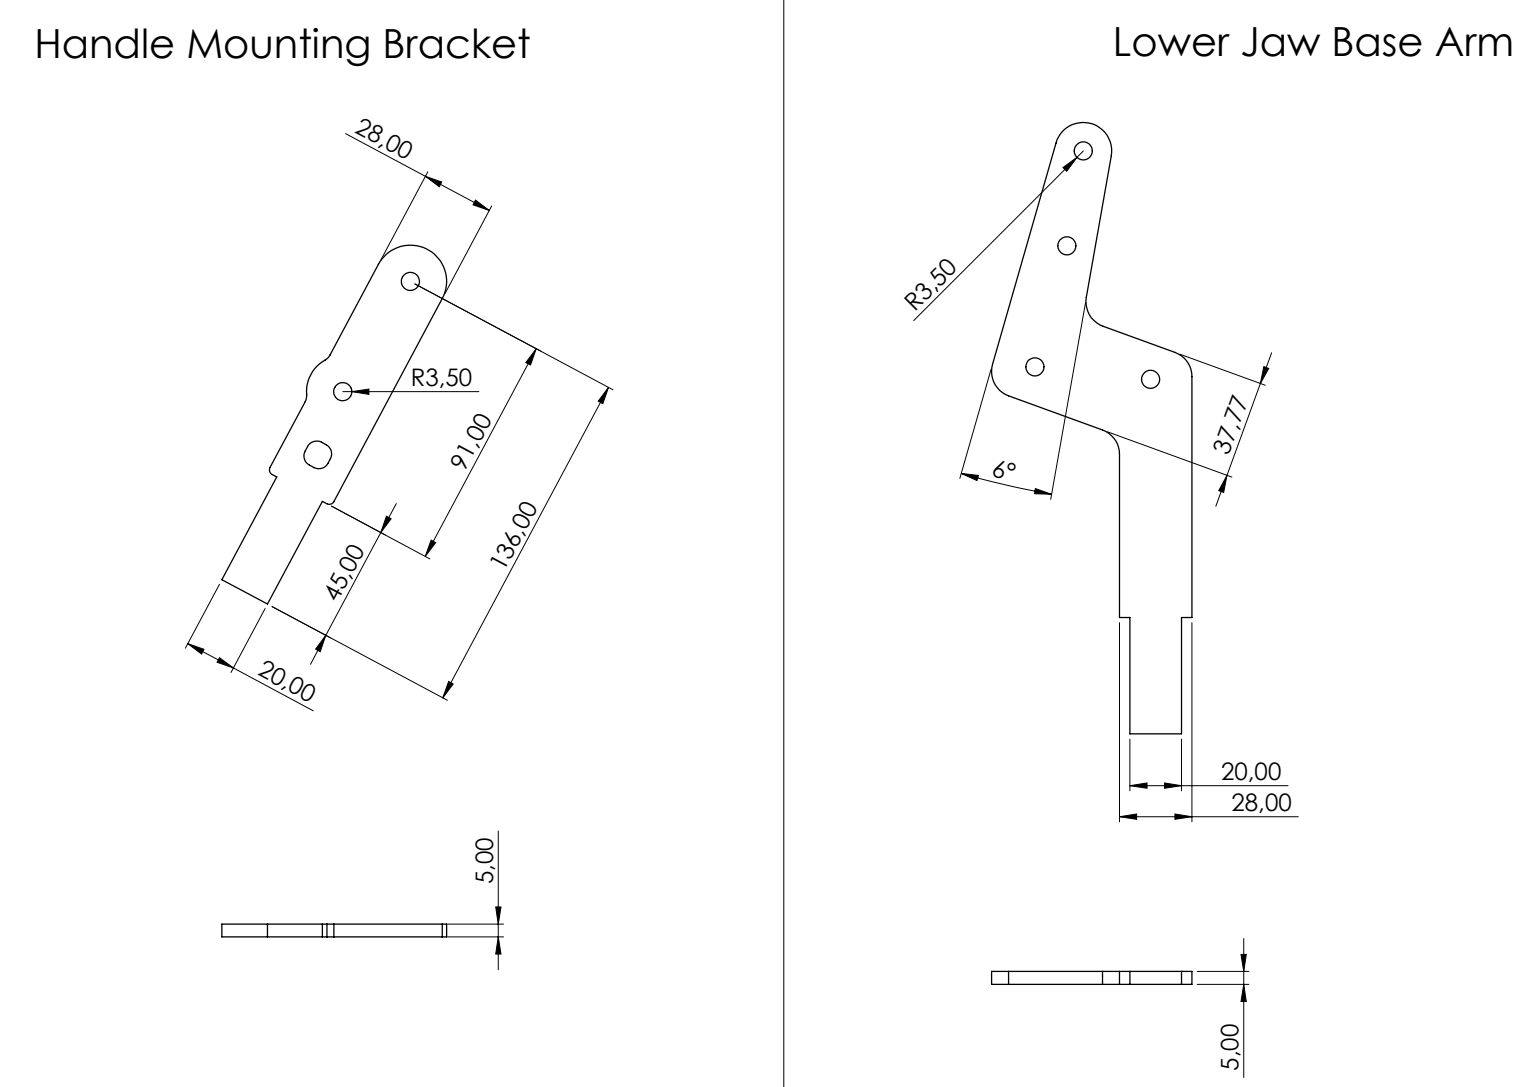
ISO-10303-21;
HEADER;
FILE_DESCRIPTION (('STEP AP214'),
    '1' );
FILE_NAME ('Handle Mounting Bracket.step',
    '2026-10-06T08:24:18',
    ( '' ),
    ( '' ),
    'SwSTEP 2.0',
    'SolidWorks 2020',
    '' );
FILE_SCHEMA (( 'AUTOMOTIVE_DESIGN' ));
ENDSEC;

DATA;
#12=AXIS2_PLACEMENT_3D ( 'NONE', #3802, #4074, #7998 ) ;
#21=PLANE ( 'NONE',  #9517 ) ;
#25=AXIS2_PLACEMENT_3D ( 'NONE', #9737, #2431, #8928 ) ;
#36=EDGE_CURVE ( 'NONE', #6471, #8445, #5902, .T. ) ;
#38=ORIENTED_EDGE ( 'NONE', *, *, #7830, .T. ) ;
#56=VERTEX_POINT ( 'NONE', #5109 ) ;
#58=CARTESIAN_POINT ( 'NONE',  ( -101.0297452788102817, -7.500000000000000000, -342.4231267849074811 ) ) ;
#62=ORIENTED_EDGE ( 'NONE', *, *, #1562, .F. ) ;
#65=DIRECTION ( 'NONE',  ( -0.8820010751365716661, 0.000000000000000000, -0.4712473909295749053 ) ) ;
#66=CARTESIAN_POINT ( 'NONE',  ( -87.43749534091338660, -7.500000000000000000, -367.8627987905216514 ) ) ;
#77=VECTOR ( 'NONE', #6835, 1000.000000000000000 ) ;
#85=DIRECTION ( 'NONE',  ( 0.000000000000000000, -1.000000000000000000, 0.000000000000000000 ) ) ;
#86=VECTOR ( 'NONE', #9017, 1000.000000000000000 ) ;
#96=CARTESIAN_POINT ( 'NONE',  ( -102.0103468492230547, -7.500000000000000000, -289.6591388711787545 ) ) ;
#120=CARTESIAN_POINT ( 'NONE',  ( -77.67426137820133647, -2.500000000000000000, -345.8174414091573681 ) ) ;
#132=DIRECTION ( 'NONE',  ( -0.4712473909295827323, 0.000000000000000000, 0.8820010751365675583 ) ) ;
#186=EDGE_LOOP ( 'NONE', ( #828, #1603, #62, #6851 ) ) ;
#211=VECTOR ( 'NONE', #3924, 1000.000000000000000 ) ;
#216=DIRECTION ( 'NONE',  ( 0.4712473909295827323, 0.000000000000000000, -0.8820010751365675583 ) ) ;
#230=LINE ( 'NONE', #8685, #4617 ) ;
#241=DIRECTION ( 'NONE',  ( 0.8820010751365678914, 0.000000000000000000, 0.4712473909295818442 ) ) ;
#251=CIRCLE ( 'NONE', #9352, 3.500000000000003997 ) ;
#257=ORIENTED_EDGE ( 'NONE', *, *, #493, .F. ) ;
#269=VERTEX_POINT ( 'NONE', #6973 ) ;
#290=CARTESIAN_POINT ( 'NONE',  ( -59.08872748607741698, -7.500000000000000000, -420.9212224720619702 ) ) ;
#304=ORIENTED_EDGE ( 'NONE', *, *, #2921, .F. ) ;
#306=VERTEX_POINT ( 'NONE', #406 ) ;
#316=AXIS2_PLACEMENT_3D ( 'NONE', #10425, #6337, #7104 ) ;
#320=VERTEX_POINT ( 'NONE', #10191 ) ;
#324=CARTESIAN_POINT ( 'NONE',  ( -99.26574312853713877, -7.500000000000000000, -341.4806320030483562 ) ) ;
#354=ORIENTED_EDGE ( 'NONE', *, *, #10397, .T. ) ;
#363=EDGE_CURVE ( 'NONE', #1218, #8202, #3035, .T. ) ;
#389=AXIS2_PLACEMENT_3D ( 'NONE', #10091, #3429, #953 ) ;
#390=ORIENTED_EDGE ( 'NONE', *, *, #6600, .F. ) ;
#392=CARTESIAN_POINT ( 'NONE',  ( -79.04021210711869116, -7.500000000000000000, -328.4066924704651456 ) ) ;
#393=CARTESIAN_POINT ( 'NONE',  ( -77.77979771402830522, -2.500000000000000000, -385.9384419754180158 ) ) ;
#394=ORIENTED_EDGE ( 'NONE', *, *, #6640, .T. ) ;
#404=DIRECTION ( 'NONE',  ( 0.000000000000000000, -1.000000000000000000, 0.000000000000000000 ) ) ;
#406=CARTESIAN_POINT ( 'NONE',  ( -79.74686404004059170, -2.500000000000000000, -383.9321052860355508 ) ) ;
#416=ORIENTED_EDGE ( 'NONE', *, *, #9414, .F. ) ;
#422=EDGE_CURVE ( 'NONE', #306, #9067, #9592, .T. ) ;
#425=CARTESIAN_POINT ( 'NONE',  ( -84.02975002432511076, -2.500000000000000000, -342.4104245220563030 ) ) ;
#426=AXIS2_PLACEMENT_3D ( 'NONE', #4824, #7296, #1375 ) ;
#432=EDGE_CURVE ( 'NONE', #700, #6716, #7233, .T. ) ;
#437=EDGE_CURVE ( 'NONE', #3828, #7650, #10190, .T. ) ;
#465=( LENGTH_UNIT ( ) NAMED_UNIT ( * ) SI_UNIT ( .MILLI., .METRE. ) );
#473=ORIENTED_EDGE ( 'NONE', *, *, #1711, .T. ) ;
#474=CIRCLE ( 'NONE', #7341, 4.000000000000008882 ) ;
#476=CARTESIAN_POINT ( 'NONE',  ( -78.61675616006050404, -7.500000000000000000, -344.0534392588842252 ) ) ;
#486=CARTESIAN_POINT ( 'NONE',  ( -79.74686404004059170, -7.500000000000000000, -383.9321052860355508 ) ) ;
#493=EDGE_CURVE ( 'NONE', #7563, #4961, #4707, .T. ) ;
#509=EDGE_LOOP ( 'NONE', ( #4732, #10118, #10336, #1157 ) ) ;
#512=AXIS2_PLACEMENT_3D ( 'NONE', #1643, #10610, #2448 ) ;
#520=AXIS2_PLACEMENT_3D ( 'NONE', #3309, #8355, #7553 ) ;
#529=CIRCLE ( 'NONE', #6531, 14.00000000000000888 ) ;
#531=STYLED_ITEM ( 'NONE', ( #3235 ), #1856 ) ;
#532=LINE ( 'NONE', #2793, #8706 ) ;
#536=CARTESIAN_POINT ( 'NONE',  ( -86.49427212956700828, -7.500000000000000000, -350.5299153184531633 ) ) ;
#568=EDGE_CURVE ( 'NONE', #9067, #6664, #8056, .T. ) ;
#581=VECTOR ( 'NONE', #10244, 1000.000000000000000 ) ;
#592=CIRCLE ( 'NONE', #7969, 4.000000000000009770 ) ;
#594=DIRECTION ( 'NONE',  ( 0.000000000000000000, 1.000000000000000000, -0.000000000000000000 ) ) ;
#636=CARTESIAN_POINT ( 'NONE',  ( -72.90663470096859555, -2.500000000000000000, -371.7168990827444190 ) ) ;
#640=FACE_BOUND ( 'NONE', #5175, .T. ) ;
#665=CARTESIAN_POINT ( 'NONE',  ( -79.31727611502927289, -2.500000000000000000, -351.2304352734219606 ) ) ;
#667=PRODUCT_DEFINITION_CONTEXT ( 'detailed design', #7443, 'design' ) ;
#670=EDGE_CURVE ( 'NONE', #1738, #2124, #8074, .T. ) ;
#681=CIRCLE ( 'NONE', #10112, 3.499999999999997335 ) ;
#696=CYLINDRICAL_SURFACE ( 'NONE', #389, 1.999999999999980238 ) ;
#700=VERTEX_POINT ( 'NONE', #818 ) ;
#703=DIRECTION ( 'NONE',  ( -0.4712473909295803454, 0.000000000000000000, 0.8820010751365688906 ) ) ;
#709=CARTESIAN_POINT ( 'NONE',  ( -119.6503683519543983, -2.500000000000000000, -299.0840866897705155 ) ) ;
#713=( LENGTH_UNIT ( ) NAMED_UNIT ( * ) SI_UNIT ( .MILLI., .METRE. ) );
#730=DIRECTION ( 'NONE',  ( 0.4712473909295803454, 0.000000000000000000, -0.8820010751365688906 ) ) ;
#750=ORIENTED_EDGE ( 'NONE', *, *, #4566, .F. ) ;
#751=ORIENTED_EDGE ( 'NONE', *, *, #437, .F. ) ;
#773=DIRECTION ( 'NONE',  ( 0.000000000000000000, 1.000000000000000000, -0.000000000000000000 ) ) ;
#778=ORIENTED_EDGE ( 'NONE', *, *, #2712, .F. ) ;
#789=FACE_OUTER_BOUND ( 'NONE', #10203, .T. ) ;
#795=CARTESIAN_POINT ( 'NONE',  ( -72.90663470096859555, -2.500000000000000000, -371.7168990827444190 ) ) ;
#803=ORIENTED_EDGE ( 'NONE', *, *, #2276, .T. ) ;
#807=CARTESIAN_POINT ( 'NONE',  ( -98.44423576012317767, -2.500000000000000000, -338.7741350709160315 ) ) ;
#812=CARTESIAN_POINT ( 'NONE',  ( -76.33371517498638070, -2.500000000000000000, -329.2281998388791635 ) ) ;
#818=CARTESIAN_POINT ( 'NONE',  ( -87.43749534091338660, -2.500000000000000000, -367.8627987905216514 ) ) ;
#826=EDGE_LOOP ( 'NONE', ( #4070, #3945, #7397, #4001, #5011, #9817, #8400, #8877 ) ) ;
#828=ORIENTED_EDGE ( 'NONE', *, *, #8175, .T. ) ;
#862=DIRECTION ( 'NONE',  ( 0.8820010751365675583, 0.000000000000000000, 0.4712473909295827323 ) ) ;
#875=ORIENTED_EDGE ( 'NONE', *, *, #1881, .F. ) ;
#889=DIRECTION ( 'NONE',  ( 0.000000000000000000, -1.000000000000000000, 0.000000000000000000 ) ) ;
#895=CYLINDRICAL_SURFACE ( 'NONE', #7546, 13.99999999999999645 ) ;
#902=DIRECTION ( 'NONE',  ( -0.4712473909295827323, 0.000000000000000000, 0.8820010751365675583 ) ) ;
#912=LINE ( 'NONE', #4202, #6782 ) ;
#916=DIRECTION ( 'NONE',  ( 0.000000000000000000, 1.000000000000000000, -0.000000000000000000 ) ) ;
#932=VERTEX_POINT ( 'NONE', #9124 ) ;
#946=ORIENTED_EDGE ( 'NONE', *, *, #9826, .T. ) ;
#948=DIRECTION ( 'NONE',  ( 0.000000000000000000, -1.000000000000000000, 0.000000000000000000 ) ) ;
#953=DIRECTION ( 'NONE',  ( -0.4712473909295860630, 0.000000000000000000, 0.8820010751365656709 ) ) ;
#968=DIRECTION ( 'NONE',  ( 0.000000000000000000, 1.000000000000000000, -0.000000000000000000 ) ) ;
#974=CARTESIAN_POINT ( 'NONE',  ( -46.74071243416547361, -2.500000000000000000, -414.3237589990478114 ) ) ;
#977=EDGE_CURVE ( 'NONE', #5188, #932, #681, .T. ) ;
#1011=DIRECTION ( 'NONE',  ( 0.8820010751365716661, 0.000000000000000000, 0.4712473909295749053 ) ) ;
#1034=CARTESIAN_POINT ( 'NONE',  ( -72.90663470096859555, -7.500000000000000000, -371.7168990827444190 ) ) ;
#1035=AXIS2_PLACEMENT_3D ( 'NONE', #974, #1730, #862 ) ;
#1040=AXIS2_PLACEMENT_3D ( 'NONE', #7215, #5321, #6238 ) ;
#1048=ORIENTED_EDGE ( 'NONE', *, *, #5342, .F. ) ;
#1052=VERTEX_POINT ( 'NONE', #6047 ) ;
#1093=CIRCLE ( 'NONE', #4515, 5.000000000000008882 ) ;
#1106=CARTESIAN_POINT ( 'NONE',  ( -82.18980308971114823, -2.500000000000000000, -388.2946789300659134 ) ) ;
#1119=ORIENTED_EDGE ( 'NONE', *, *, #7066, .F. ) ;
#1126=LINE ( 'NONE', #2795, #10298 ) ;
#1128=CARTESIAN_POINT ( 'NONE',  ( -72.90663470096859555, -7.500000000000000000, -371.7168990827444190 ) ) ;
#1140=ORIENTED_EDGE ( 'NONE', *, *, #4953, .T. ) ;
#1152=ORIENTED_EDGE ( 'NONE', *, *, #4382, .T. ) ;
#1157=ORIENTED_EDGE ( 'NONE', *, *, #2791, .F. ) ;
#1167=CIRCLE ( 'NONE', #7689, 5.000000000000006217 ) ;
#1170=ORIENTED_EDGE ( 'NONE', *, *, #2276, .F. ) ;
#1177=FACE_OUTER_BOUND ( 'NONE', #10616, .T. ) ;
#1190=CARTESIAN_POINT ( 'NONE',  ( -89.32175647514451100, -2.500000000000000000, -345.2379088676337915 ) ) ;
#1197=LINE ( 'NONE', #8604, #4995 ) ;
#1200=CARTESIAN_POINT ( 'NONE',  ( -79.31727611502927289, -7.500000000000000000, -351.2304352734219606 ) ) ;
#1211=LINE ( 'NONE', #10139, #9926 ) ;
#1218=VERTEX_POINT ( 'NONE', #6075 ) ;
#1221=DIRECTION ( 'NONE',  ( 0.000000000000000000, 1.000000000000000000, -0.000000000000000000 ) ) ;
#1257=ORIENTED_EDGE ( 'NONE', *, *, #2987, .F. ) ;
#1266=AXIS2_PLACEMENT_3D ( 'NONE', #9096, #5703, #2433 ) ;
#1276=AXIS2_PLACEMENT_3D ( 'NONE', #6620, #9898, #9257 ) ;
#1286=PLANE ( 'NONE',  #4156 ) ;
#1301=VERTEX_POINT ( 'NONE', #6124 ) ;
#1308=EDGE_LOOP ( 'NONE', ( #7865, #5755, #3971, #875 ) ) ;
#1317=CARTESIAN_POINT ( 'NONE',  ( -34.39269738225353024, -2.500000000000000000, -407.7262955260336525 ) ) ;
#1327=FACE_OUTER_BOUND ( 'NONE', #5253, .T. ) ;
#1341=CARTESIAN_POINT ( 'NONE',  ( -119.6503683519543983, -7.500000000000000000, -299.0840866897705155 ) ) ;
#1344=CARTESIAN_POINT ( 'NONE',  ( -78.52752440735136474, -2.500000000000000000, -384.5389737553005034 ) ) ;
#1351=DIRECTION ( 'NONE',  ( -0.8820010751365675583, 0.000000000000000000, -0.4712473909295827323 ) ) ;
#1361=AXIS2_PLACEMENT_3D ( 'NONE', #9213, #7589, #5809 ) ;
#1363=ORIENTED_EDGE ( 'NONE', *, *, #977, .T. ) ;
#1364=CARTESIAN_POINT ( 'NONE',  ( -79.31727611502927289, -2.500000000000000000, -351.2304352734219606 ) ) ;
#1373=VERTEX_POINT ( 'NONE', #1341 ) ;
#1375=DIRECTION ( 'NONE',  ( -0.8820010751365678914, 0.000000000000000000, -0.4712473909295818442 ) ) ;
#1380=CARTESIAN_POINT ( 'NONE',  ( -86.86306229143158930, -2.500000000000000000, -370.6132103076870976 ) ) ;
#1384=FACE_OUTER_BOUND ( 'NONE', #4703, .T. ) ;
#1418=VERTEX_POINT ( 'NONE', #6174 ) ;
#1424=CARTESIAN_POINT ( 'NONE',  ( -80.80421425739181984, -2.500000000000000000, -329.3491872523243842 ) ) ;
#1429=ORIENTED_EDGE ( 'NONE', *, *, #5752, .F. ) ;
#1432=ORIENTED_EDGE ( 'NONE', *, *, #6163, .F. ) ;
#1457=AXIS2_PLACEMENT_3D ( 'NONE', #5077, #10617, #4173 ) ;
#1460=PRODUCT_CONTEXT ( 'NONE', #2761, 'mechanical' ) ;
#1467=ORIENTED_EDGE ( 'NONE', *, *, #5835, .F. ) ;
#1477=ADVANCED_FACE ( 'NONE', ( #4789 ), #7258, .F. ) ;
#1480=DIRECTION ( 'NONE',  ( -0.8820010751365675583, 0.000000000000000000, -0.4712473909295827323 ) ) ;
#1481=ORIENTED_EDGE ( 'NONE', *, *, #1562, .T. ) ;
#1485=ADVANCED_FACE ( 'NONE', ( #9729 ), #3975, .T. ) ;
#1493=ORIENTED_EDGE ( 'NONE', *, *, #432, .F. ) ;
#1514=CARTESIAN_POINT ( 'NONE',  ( -84.02975002432511076, -2.500000000000000000, -342.4104245220563030 ) ) ;
#1519=VERTEX_POINT ( 'NONE', #9321 ) ;
#1525=EDGE_LOOP ( 'NONE', ( #4822, #7801, #3032, #3409 ) ) ;
#1535=ADVANCED_FACE ( 'NONE', ( #10169 ), #9270, .T. ) ;
#1547=CARTESIAN_POINT ( 'NONE',  ( -80.80421425739181984, -7.500000000000000000, -329.3491872523243842 ) ) ;
#1549=VECTOR ( 'NONE', #3392, 1000.000000000000000 ) ;
#1561=ORIENTED_EDGE ( 'NONE', *, *, #568, .T. ) ;
#1562=EDGE_CURVE ( 'NONE', #320, #8561, #2812, .T. ) ;
#1593=VECTOR ( 'NONE', #8757, 1000.000000000000000 ) ;
#1603=ORIENTED_EDGE ( 'NONE', *, *, #9616, .T. ) ;
#1607=CARTESIAN_POINT ( 'NONE',  ( -83.90876261087991850, -7.500000000000000000, -346.8809236044617137 ) ) ;
#1619=PLANE ( 'NONE',  #3401 ) ;
#1625=( NAMED_UNIT ( * ) PLANE_ANGLE_UNIT ( ) SI_UNIT ( $, .RADIAN. ) );
#1630=VECTOR ( 'NONE', #3515, 1000.000000000000000 ) ;
#1631=CIRCLE ( 'NONE', #1276, 5.000000000000008882 ) ;
#1643=CARTESIAN_POINT ( 'NONE',  ( -82.18980308971114823, -7.500000000000000000, -388.2946789300659134 ) ) ;
#1671=EDGE_CURVE ( 'NONE', #9606, #10567, #2305, .T. ) ;
#1677=ORIENTED_EDGE ( 'NONE', *, *, #10150, .F. ) ;
#1685=CYLINDRICAL_SURFACE ( 'NONE', #3076, 1.999999999999998224 ) ;
#1689=VERTEX_POINT ( 'NONE', #3721 ) ;
#1701=CARTESIAN_POINT ( 'NONE',  ( -82.14476046060677561, -2.500000000000000000, -345.9384288226025888 ) ) ;
#1702=CARTESIAN_POINT ( 'NONE',  ( -69.81963093799060971, -7.500000000000000000, -370.0675332144908793 ) ) ;
#1711=EDGE_CURVE ( 'NONE', #4107, #7563, #6183, .T. ) ;
#1718=CARTESIAN_POINT ( 'NONE',  ( -78.09771732525952359, -7.500000000000000000, -330.1706946207383453 ) ) ;
#1729=SURFACE_SIDE_STYLE ('',( #3344 ) ) ;
#1730=DIRECTION ( 'NONE',  ( 0.000000000000000000, 1.000000000000000000, -0.000000000000000000 ) ) ;
#1738=VERTEX_POINT ( 'NONE', #7855 ) ;
#1749=CARTESIAN_POINT ( 'NONE',  ( -34.39269738225353024, -7.500000000000000000, -407.7262955260336525 ) ) ;
#1751=CYLINDRICAL_SURFACE ( 'NONE', #1457, 3.499999999999997335 ) ;
#1755=CIRCLE ( 'NONE', #3123, 3.500000000000003997 ) ;
#1757=CARTESIAN_POINT ( 'NONE',  ( -34.39269738225353024, -2.500000000000000000, -407.7262955260336525 ) ) ;
#1765=VECTOR ( 'NONE', #5247, 1000.000000000000000 ) ;
#1774=EDGE_CURVE ( 'NONE', #9600, #5739, #2422, .T. ) ;
#1799=CIRCLE ( 'NONE', #4031, 14.00000000000000888 ) ;
#1804=AXIS2_PLACEMENT_3D ( 'NONE', #6758, #9066, #9923 ) ;
#1814=ORIENTED_EDGE ( 'NONE', *, *, #6930, .T. ) ;
#1818=DIRECTION ( 'NONE',  ( -0.8820010751365675583, 0.000000000000000000, -0.4712473909295825103 ) ) ;
#1822=CARTESIAN_POINT ( 'NONE',  ( -119.6503683519543983, -2.500000000000000000, -299.0840866897705155 ) ) ;
#1847=ORIENTED_EDGE ( 'NONE', *, *, #7977, .F. ) ;
#1856=MANIFOLD_SOLID_BREP ( 'Stock-MAS-686-1', #5554 ) ;
#1869=EDGE_CURVE ( 'NONE', #932, #4003, #7480, .T. ) ;
#1874=DIRECTION ( 'NONE',  ( 0.000000000000000000, 1.000000000000000000, -0.000000000000000000 ) ) ;
#1881=EDGE_CURVE ( 'NONE', #1689, #1519, #4653, .T. ) ;
#1897=FACE_OUTER_BOUND ( 'NONE', #2231, .T. ) ;
#1911=LINE ( 'NONE', #5984, #3303 ) ;
#1915=DIRECTION ( 'NONE',  ( 0.000000000000000000, -1.000000000000000000, 0.000000000000000000 ) ) ;
#1919=DIRECTION ( 'NONE',  ( 0.000000000000000000, 1.000000000000000000, -0.000000000000000000 ) ) ;
#1943=ADVANCED_FACE ( 'NONE', ( #2115 ), #6140, .F. ) ;
#1950=UNCERTAINTY_MEASURE_WITH_UNIT (LENGTH_MEASURE( 1.000000000000000082E-05 ), #10396, 'distance_accuracy_value', 'NONE');
#1979=LINE ( 'NONE', #6154, #1765 ) ;
#1995=EDGE_CURVE ( 'NONE', #1689, #8136, #1197, .T. ) ;
#2061=AXIS2_PLACEMENT_3D ( 'NONE', #6419, #7392, #730 ) ;
#2064=CIRCLE ( 'NONE', #1035, 3.499999999999997335 ) ;
#2077=FILL_AREA_STYLE ('',( #4544 ) ) ;
#2082=EDGE_CURVE ( 'NONE', #56, #4107, #2972, .T. ) ;
#2084=ORIENTED_EDGE ( 'NONE', *, *, #8293, .F. ) ;
#2089=DIRECTION ( 'NONE',  ( -0.4712473909295860630, 0.000000000000000000, 0.8820010751365656709 ) ) ;
#2103=CARTESIAN_POINT ( 'NONE',  ( -80.80421425739181984, -2.500000000000000000, -329.3491872523243842 ) ) ;
#2115=FACE_OUTER_BOUND ( 'NONE', #7123, .T. ) ;
#2117=ORIENTED_EDGE ( 'NONE', *, *, #1671, .F. ) ;
#2124=VERTEX_POINT ( 'NONE', #5758 ) ;
#2166=ORIENTED_EDGE ( 'NONE', *, *, #7924, .T. ) ;
#2177=ORIENTED_EDGE ( 'NONE', *, *, #2731, .F. ) ;
#2192=DIRECTION ( 'NONE',  ( 0.4712473909295827323, 0.000000000000000000, -0.8820010751365675583 ) ) ;
#2209=CARTESIAN_POINT ( 'NONE',  ( -102.0103468492230547, -2.500000000000000000, -289.6591388711787545 ) ) ;
#2222=CIRCLE ( 'NONE', #6884, 4.000000000000009770 ) ;
#2231=EDGE_LOOP ( 'NONE', ( #5461, #1677, #4432, #9762 ) ) ;
#2261=DIRECTION ( 'NONE',  ( -0.8820010751365675583, 0.000000000000000000, -0.4712473909295827323 ) ) ;
#2267=CIRCLE ( 'NONE', #8270, 3.499999999999997335 ) ;
#2276=EDGE_CURVE ( 'NONE', #8515, #5739, #3659, .T. ) ;
#2284=CARTESIAN_POINT ( 'NONE',  ( -72.90663470096859555, -2.500000000000000000, -371.7168990827444190 ) ) ;
#2302=CARTESIAN_POINT ( 'NONE',  ( -46.74071243416547361, -7.500000000000000000, -414.3237589990478114 ) ) ;
#2305=CIRCLE ( 'NONE', #1040, 3.500000000000003997 ) ;
#2340=ORIENTED_EDGE ( 'NONE', *, *, #36, .F. ) ;
#2350=LINE ( 'NONE', #8952, #5308 ) ;
#2353=EDGE_CURVE ( 'NONE', #56, #5548, #474, .T. ) ;
#2363=FACE_OUTER_BOUND ( 'NONE', #186, .T. ) ;
#2370=CARTESIAN_POINT ( 'NONE',  ( -34.39269738225353024, -2.500000000000000000, -407.7262955260336525 ) ) ;
#2422=CIRCLE ( 'NONE', #7053, 1.999999999999998224 ) ;
#2431=DIRECTION ( 'NONE',  ( 0.000000000000000000, -1.000000000000000000, 0.000000000000000000 ) ) ;
#2433=DIRECTION ( 'NONE',  ( -0.8820010751365675583, 0.000000000000000000, -0.4712473909295825103 ) ) ;
#2448=DIRECTION ( 'NONE',  ( 0.4885878099338311631, 0.000000000000000000, 0.8725147288063752615 ) ) ;
#2460=LINE ( 'NONE', #96, #9501 ) ;
#2479=LINE ( 'NONE', #807, #4117 ) ;
#2497=ORIENTED_EDGE ( 'NONE', *, *, #7977, .T. ) ;
#2505=DIRECTION ( 'NONE',  ( 0.8820010751365653379, 0.000000000000000000, 0.4712473909295871732 ) ) ;
#2527=ORIENTED_EDGE ( 'NONE', *, *, #6205, .T. ) ;
#2561=ORIENTED_EDGE ( 'NONE', *, *, #1869, .F. ) ;
#2565=DIRECTION ( 'NONE',  ( 0.000000000000000000, -1.000000000000000000, 0.000000000000000000 ) ) ;
#2567=VECTOR ( 'NONE', #5886, 1000.000000000000000 ) ;
#2570=FACE_OUTER_BOUND ( 'NONE', #1525, .T. ) ;
#2573=CARTESIAN_POINT ( 'NONE',  ( -43.65370867118748777, -7.500000000000000000, -412.6743931307942717 ) ) ;
#2575=ADVANCED_FACE ( 'NONE', ( #9730, #3928, #7207, #6557 ), #1619, .F. ) ;
#2588=DIRECTION ( 'NONE',  ( -0.4712473909295827323, 0.000000000000000000, 0.8820010751365675583 ) ) ;
#2599=CARTESIAN_POINT ( 'NONE',  ( -77.67426137820133647, -7.500000000000000000, -345.8174414091573681 ) ) ;
#2607=VERTEX_POINT ( 'NONE', #58 ) ;
#2615=ORIENTED_EDGE ( 'NONE', *, *, #4909, .T. ) ;
#2644=VECTOR ( 'NONE', #4287, 1000.000000000000000 ) ;
#2657=FACE_OUTER_BOUND ( 'NONE', #6360, .T. ) ;
#2669=VECTOR ( 'NONE', #5090, 1000.000000000000000 ) ;
#2671=ORIENTED_EDGE ( 'NONE', *, *, #9703, .T. ) ;
#2686=LINE ( 'NONE', #5037, #10175 ) ;
#2689=ORIENTED_EDGE ( 'NONE', *, *, #2987, .T. ) ;
#2694=LINE ( 'NONE', #6012, #1549 ) ;
#2698=EDGE_CURVE ( 'NONE', #8515, #2607, #8883, .T. ) ;
#2704=CARTESIAN_POINT ( 'NONE',  ( -78.61675616006050404, -2.500000000000000000, -344.0534392588842252 ) ) ;
#2712=EDGE_CURVE ( 'NONE', #9606, #7707, #9555, .T. ) ;
#2731=EDGE_CURVE ( 'NONE', #8080, #700, #1167, .T. ) ;
#2761=APPLICATION_CONTEXT ( 'automotive_design' ) ;
#2791=EDGE_CURVE ( 'NONE', #3089, #6862, #532, .T. ) ;
#2793=CARTESIAN_POINT ( 'NONE',  ( -78.61675616006050404, -2.500000000000000000, -344.0534392588842252 ) ) ;
#2795=CARTESIAN_POINT ( 'NONE',  ( -76.33371517498638070, -7.500000000000000000, -329.2281998388791635 ) ) ;
#2812=LINE ( 'NONE', #392, #3333 ) ;
#2817=AXIS2_PLACEMENT_3D ( 'NONE', #8634, #3966, #3161 ) ;
#2820=AXIS2_PLACEMENT_3D ( 'NONE', #2370, #3173, #8866 ) ;
#2821=CARTESIAN_POINT ( 'NONE',  ( -49.82771619714345235, -2.500000000000000000, -415.9731248673013511 ) ) ;
#2826=CARTESIAN_POINT ( 'NONE',  ( -59.08872748607741698, -2.500000000000000000, -420.9212224720619702 ) ) ;
#2853=CARTESIAN_POINT ( 'NONE',  ( -75.78927181448300132, -2.500000000000000000, -349.3454457097035970 ) ) ;
#2858=FACE_OUTER_BOUND ( 'NONE', #7879, .T. ) ;
#2862=ORIENTED_EDGE ( 'NONE', *, *, #9957, .F. ) ;
#2865=DIRECTION ( 'NONE',  ( -0.4712473909295803454, 0.000000000000000000, 0.8820010751365688906 ) ) ;
#2874=VERTEX_POINT ( 'NONE', #3748 ) ;
#2877=DIRECTION ( 'NONE',  ( 0.000000000000000000, -1.000000000000000000, 0.000000000000000000 ) ) ;
#2878=ORIENTED_EDGE ( 'NONE', *, *, #422, .F. ) ;
#2906=ORIENTED_EDGE ( 'NONE', *, *, #6007, .F. ) ;
#2914=CYLINDRICAL_SURFACE ( 'NONE', #8484, 3.500000000000003997 ) ;
#2917=ORIENTED_EDGE ( 'NONE', *, *, #6163, .T. ) ;
#2921=EDGE_CURVE ( 'NONE', #320, #8575, #6870, .T. ) ;
#2932=DIRECTION ( 'NONE',  ( 0.8820010751365675583, 0.000000000000000000, 0.4712473909295827323 ) ) ;
#2940=ORIENTED_EDGE ( 'NONE', *, *, #9101, .T. ) ;
#2946=PLANE ( 'NONE',  #6232 ) ;
#2972=LINE ( 'NONE', #665, #5437 ) ;
#2974=ORIENTED_EDGE ( 'NONE', *, *, #6930, .F. ) ;
#2987=EDGE_CURVE ( 'NONE', #8626, #7650, #1211, .T. ) ;
#2996=DIRECTION ( 'NONE',  ( 0.000000000000000000, -1.000000000000000000, 0.000000000000000000 ) ) ;
#2998=EDGE_CURVE ( 'NONE', #4191, #5439, #5397, .T. ) ;
#3002=CARTESIAN_POINT ( 'NONE',  ( -91.84750071659622961, -2.366295999999999733, -370.2190357451694922 ) ) ;
#3017=CARTESIAN_POINT ( 'NONE',  ( -79.04021210711869116, -2.500000000000000000, -328.4066924704651456 ) ) ;
#3021=ORIENTED_EDGE ( 'NONE', *, *, #6600, .T. ) ;
#3032=ORIENTED_EDGE ( 'NONE', *, *, #7790, .F. ) ;
#3035=LINE ( 'NONE', #1424, #7979 ) ;
#3059=DIRECTION ( 'NONE',  ( 0.000000000000000000, 1.000000000000000000, -0.000000000000000000 ) ) ;
#3076=AXIS2_PLACEMENT_3D ( 'NONE', #8078, #773, #7383 ) ;
#3089=VERTEX_POINT ( 'NONE', #2704 ) ;
#3091=( NAMED_UNIT ( * ) PLANE_ANGLE_UNIT ( ) SI_UNIT ( $, .RADIAN. ) );
#3094=VERTEX_POINT ( 'NONE', #2599 ) ;
#3113=ADVANCED_FACE ( 'NONE', ( #1897 ), #5367, .T. ) ;
#3121=ADVANCED_FACE ( 'NONE', ( #4682 ), #10373, .T. ) ;
#3123=AXIS2_PLACEMENT_3D ( 'NONE', #2284, #3198, #8776 ) ;
#3161=DIRECTION ( 'NONE',  ( 1.000000000000000000, 0.000000000000000000, 0.000000000000000000 ) ) ;
#3170=LINE ( 'NONE', #6444, #211 ) ;
#3171=VECTOR ( 'NONE', #7340, 1000.000000000000000 ) ;
#3173=DIRECTION ( 'NONE',  ( 0.8820010751365675583, 0.000000000000000000, 0.4712473909295827323 ) ) ;
#3189=ADVANCED_FACE ( 'NONE', ( #2858 ), #4464, .T. ) ;
#3193=CARTESIAN_POINT ( 'NONE',  ( -85.79375217459825365, -7.500000000000000000, -343.3529193039154279 ) ) ;
#3198=DIRECTION ( 'NONE',  ( 0.000000000000000000, 1.000000000000000000, -0.000000000000000000 ) ) ;
#3235=PRESENTATION_STYLE_ASSIGNMENT (( #3398 ) ) ;
#3245=ORIENTED_EDGE ( 'NONE', *, *, #2698, .T. ) ;
#3247=EDGE_LOOP ( 'NONE', ( #4992, #9977, #8474, #1048 ) ) ;
#3251=EDGE_CURVE ( 'NONE', #8202, #5927, #9519, .T. ) ;
#3276=ORIENTED_EDGE ( 'NONE', *, *, #7206, .F. ) ;
#3278=DIRECTION ( 'NONE',  ( 0.000000000000000000, -1.000000000000000000, -0.000000000000000000 ) ) ;
#3285=CARTESIAN_POINT ( 'NONE',  ( -81.20226567874760804, -2.366295999999999733, -347.7024309728756748 ) ) ;
#3297=ORIENTED_EDGE ( 'NONE', *, *, #10481, .F. ) ;
#3303=VECTOR ( 'NONE', #5234, 1000.000000000000000 ) ;
#3305=PRODUCT_DEFINITION ( 'UNKNOWN', '', #6449, #667 ) ;
#3309=CARTESIAN_POINT ( 'NONE',  ( -46.74071243416547361, -7.500000000000000000, -414.3237589990478114 ) ) ;
#3318=FACE_OUTER_BOUND ( 'NONE', #10255, .T. ) ;
#3333=VECTOR ( 'NONE', #8346, 1000.000000000000000 ) ;
#3344=SURFACE_STYLE_FILL_AREA ( #5700 ) ;
#3375=LINE ( 'NONE', #9981, #2567 ) ;
#3392=DIRECTION ( 'NONE',  ( -0.4712473909295827323, 0.000000000000000000, 0.8820010751365675583 ) ) ;
#3398=SURFACE_STYLE_USAGE ( .BOTH. , #1729 ) ;
#3401=AXIS2_PLACEMENT_3D ( 'NONE', #5585, #3278, #8170 ) ;
#3409=ORIENTED_EDGE ( 'NONE', *, *, #9957, .T. ) ;
#3429=DIRECTION ( 'NONE',  ( 0.000000000000000000, 1.000000000000000000, -0.000000000000000000 ) ) ;
#3432=CARTESIAN_POINT ( 'NONE',  ( -98.44423576012317767, -7.500000000000000000, -338.7741350709160315 ) ) ;
#3434=ORIENTED_EDGE ( 'NONE', *, *, #9826, .F. ) ;
#3446=ADVANCED_FACE ( 'NONE', ( #6116 ), #5464, .F. ) ;
#3451=DIRECTION ( 'NONE',  ( 0.4712473909295803454, 0.000000000000000000, -0.8820010751365688906 ) ) ;
#3474=EDGE_LOOP ( 'NONE', ( #9966, #5789, #2878, #8887 ) ) ;
#3487=CARTESIAN_POINT ( 'NONE',  ( -84.60928256584868734, -2.500000000000000000, -354.0579196189994491 ) ) ;
#3515=DIRECTION ( 'NONE',  ( 0.4712473909295827323, 0.000000000000000000, -0.8820010751365675583 ) ) ;
#3539=ORIENTED_EDGE ( 'NONE', *, *, #7327, .F. ) ;
#3547=CARTESIAN_POINT ( 'NONE',  ( -78.61675616006050404, -2.500000000000000000, -344.0534392588842252 ) ) ;
#3563=ORIENTED_EDGE ( 'NONE', *, *, #4591, .F. ) ;
#3588=DIRECTION ( 'NONE',  ( 0.000000000000000000, -1.000000000000000000, 0.000000000000000000 ) ) ;
#3589=ADVANCED_FACE ( 'NONE', ( #10517 ), #696, .T. ) ;
#3618=ORIENTED_EDGE ( 'NONE', *, *, #4169, .F. ) ;
#3648=DIRECTION ( 'NONE',  ( 0.000000000000000000, -1.000000000000000000, 0.000000000000000000 ) ) ;
#3658=ADVANCED_FACE ( 'NONE', ( #8419 ), #8261, .T. ) ;
#3659=LINE ( 'NONE', #5476, #4420 ) ;
#3665=DIRECTION ( 'NONE',  ( 0.4712473909295827323, 0.000000000000000000, -0.8820010751365675583 ) ) ;
#3669=ADVANCED_FACE ( 'NONE', ( #9075 ), #4344, .T. ) ;
#3674=ORIENTED_EDGE ( 'NONE', *, *, #6824, .F. ) ;
#3681=DIRECTION ( 'NONE',  ( -0.8820010751365675583, 0.000000000000000000, -0.4712473909295825103 ) ) ;
#3695=ORIENTED_EDGE ( 'NONE', *, *, #4169, .T. ) ;
#3721=CARTESIAN_POINT ( 'NONE',  ( -85.79375217459825365, -2.500000000000000000, -343.3529193039154279 ) ) ;
#3731=LINE ( 'NONE', #10290, #6781 ) ;
#3734=ORIENTED_EDGE ( 'NONE', *, *, #10029, .T. ) ;
#3748=CARTESIAN_POINT ( 'NONE',  ( -76.33371517498638070, -7.500000000000000000, -329.2281998388791635 ) ) ;
#3770=ORIENTED_EDGE ( 'NONE', *, *, #10207, .T. ) ;
#3802=CARTESIAN_POINT ( 'NONE',  ( -82.96626782902075092, -2.366295999999999733, -348.6449257547347997 ) ) ;
#3805=DIRECTION ( 'NONE',  ( 0.000000000000000000, -1.000000000000000000, 0.000000000000000000 ) ) ;
#3817=AXIS2_PLACEMENT_3D ( 'NONE', #1822, #10041, #6602 ) ;
#3818=ADVANCED_FACE ( 'NONE', ( #2570 ), #5143, .T. ) ;
#3828=VERTEX_POINT ( 'NONE', #9883 ) ;
#3845=AXIS2_PLACEMENT_3D ( 'NONE', #10501, #8780, #8195 ) ;
#3871=VERTEX_POINT ( 'NONE', #6264 ) ;
#3879=DIRECTION ( 'NONE',  ( -0.8820010751365675583, 0.000000000000000000, -0.4712473909295827323 ) ) ;
#3889=DIRECTION ( 'NONE',  ( 0.000000000000000000, 1.000000000000000000, -0.000000000000000000 ) ) ;
#3893=EDGE_CURVE ( 'NONE', #1689, #7605, #1979, .T. ) ;
#3894=ORIENTED_EDGE ( 'NONE', *, *, #1995, .T. ) ;
#3899=DIRECTION ( 'NONE',  ( 0.000000000000000000, -1.000000000000000000, 0.000000000000000000 ) ) ;
#3914=ORIENTED_EDGE ( 'NONE', *, *, #36, .T. ) ;
#3916=DIRECTION ( 'NONE',  ( -0.8820010751365675583, 0.000000000000000000, -0.4712473909295827323 ) ) ;
#3924=DIRECTION ( 'NONE',  ( 0.000000000000000000, -1.000000000000000000, 0.000000000000000000 ) ) ;
#3927=EDGE_CURVE ( 'NONE', #1373, #2124, #1911, .T. ) ;
#3928=FACE_BOUND ( 'NONE', #826, .T. ) ;
#3940=AXIS2_PLACEMENT_3D ( 'NONE', #795, #2565, #9125 ) ;
#3945=ORIENTED_EDGE ( 'NONE', *, *, #6205, .F. ) ;
#3950=ORIENTED_EDGE ( 'NONE', *, *, #10074, .T. ) ;
#3953=CARTESIAN_POINT ( 'NONE',  ( -79.74686404004059170, -2.500000000000000000, -383.9321052860355508 ) ) ;
#3954=CARTESIAN_POINT ( 'NONE',  ( -75.99363846394659561, -7.500000000000000000, -373.3662649509979587 ) ) ;
#3966=DIRECTION ( 'NONE',  ( 0.000000000000000000, 0.000000000000000000, 1.000000000000000000 ) ) ;
#3971=ORIENTED_EDGE ( 'NONE', *, *, #10207, .F. ) ;
#3975=PLANE ( 'NONE',  #2820 ) ;
#4001=ORIENTED_EDGE ( 'NONE', *, *, #5951, .F. ) ;
#4003=VERTEX_POINT ( 'NONE', #2821 ) ;
#4018=DIRECTION ( 'NONE',  ( 0.000000000000000000, -1.000000000000000000, 0.000000000000000000 ) ) ;
#4031=AXIS2_PLACEMENT_3D ( 'NONE', #10563, #85, #6584 ) ;
#4042=CARTESIAN_POINT ( 'NONE',  ( -43.65370867118748777, -2.500000000000000000, -412.6743931307942717 ) ) ;
#4063=DIRECTION ( 'NONE',  ( 0.000000000000000000, -1.000000000000000000, 0.000000000000000000 ) ) ;
#4070=ORIENTED_EDGE ( 'NONE', *, *, #7641, .T. ) ;
#4072=LINE ( 'NONE', #1547, #86 ) ;
#4074=DIRECTION ( 'NONE',  ( 0.000000000000000000, -1.000000000000000000, 0.000000000000000000 ) ) ;
#4078=CARTESIAN_POINT ( 'NONE',  ( -102.0103468492230547, -2.500000000000000000, -289.6591388711787545 ) ) ;
#4082=PLANE ( 'NONE',  #9182 ) ;
#4107=VERTEX_POINT ( 'NONE', #1200 ) ;
#4117=VECTOR ( 'NONE', #3879, 1000.000000000000000 ) ;
#4156=AXIS2_PLACEMENT_3D ( 'NONE', #2853, #8692, #594 ) ;
#4163=ORIENTED_EDGE ( 'NONE', *, *, #2998, .F. ) ;
#4169=EDGE_CURVE ( 'NONE', #7605, #1418, #6411, .T. ) ;
#4173=DIRECTION ( 'NONE',  ( 0.8820010751365675583, 0.000000000000000000, 0.4712473909295827323 ) ) ;
#4191=VERTEX_POINT ( 'NONE', #8024 ) ;
#4193=ORIENTED_EDGE ( 'NONE', *, *, #6151, .F. ) ;
#4202=CARTESIAN_POINT ( 'NONE',  ( -34.39269738225353024, -7.500000000000000000, -407.7262955260336525 ) ) ;
#4204=DIRECTION ( 'NONE',  ( 0.000000000000000000, 1.000000000000000000, -0.000000000000000000 ) ) ;
#4206=( NAMED_UNIT ( * ) SI_UNIT ( $, .STERADIAN. ) SOLID_ANGLE_UNIT ( ) );
#4210=CIRCLE ( 'NONE', #10212, 4.000000000000009770 ) ;
#4234=CARTESIAN_POINT ( 'NONE',  ( -46.74071243416547361, -2.500000000000000000, -414.3237589990478114 ) ) ;
#4240=DIRECTION ( 'NONE',  ( 0.4712473909295827323, 0.000000000000000000, -0.8820010751365675583 ) ) ;
#4246=ORIENTED_EDGE ( 'NONE', *, *, #1711, .F. ) ;
#4282=ORIENTED_EDGE ( 'NONE', *, *, #6151, .T. ) ;
#4287=DIRECTION ( 'NONE',  ( 0.000000000000000000, -1.000000000000000000, 0.000000000000000000 ) ) ;
#4293=CARTESIAN_POINT ( 'NONE',  ( -80.50174572377882498, -2.500000000000000000, -340.5254349583379394 ) ) ;
#4298=ORIENTED_EDGE ( 'NONE', *, *, #432, .T. ) ;
#4305=LINE ( 'NONE', #9088, #4970 ) ;
#4308=ADVANCED_FACE ( 'NONE', ( #2363 ), #5629, .T. ) ;
#4338=CARTESIAN_POINT ( 'NONE',  ( -87.43676691142619006, -7.500000000000000000, -348.7659131681800773 ) ) ;
#4344=PLANE ( 'NONE',  #4501 ) ;
#4382=EDGE_CURVE ( 'NONE', #1301, #1519, #2686, .T. ) ;
#4403=ORIENTED_EDGE ( 'NONE', *, *, #8507, .F. ) ;
#4420=VECTOR ( 'NONE', #6286, 1000.000000000000000 ) ;
#4432=ORIENTED_EDGE ( 'NONE', *, *, #3251, .F. ) ;
#4457=CYLINDRICAL_SURFACE ( 'NONE', #10545, 3.500000000000003997 ) ;
#4464=PLANE ( 'NONE',  #5970 ) ;
#4501=AXIS2_PLACEMENT_3D ( 'NONE', #3487, #9294, #7407 ) ;
#4504=DIRECTION ( 'NONE',  ( 0.000000000000000000, 1.000000000000000000, -0.000000000000000000 ) ) ;
#4506=DIRECTION ( 'NONE',  ( 0.000000000000000000, 1.000000000000000000, -0.000000000000000000 ) ) ;
#4515=AXIS2_PLACEMENT_3D ( 'NONE', #1106, #404, #8516 ) ;
#4534=ORIENTED_EDGE ( 'NONE', *, *, #6713, .F. ) ;
#4541=VECTOR ( 'NONE', #9014, 1000.000000000000000 ) ;
#4544=FILL_AREA_STYLE_COLOUR ( '', #6096 ) ;
#4555=STYLED_ITEM ( 'NONE', ( #8676 ), #9043 ) ;
#4556=ORIENTED_EDGE ( 'NONE', *, *, #437, .T. ) ;
#4566=EDGE_CURVE ( 'NONE', #10567, #269, #4919, .T. ) ;
#4572=DIRECTION ( 'NONE',  ( 0.000000000000000000, -1.000000000000000000, 0.000000000000000000 ) ) ;
#4590=DIRECTION ( 'NONE',  ( 0.4712473909295827323, 0.000000000000000000, -0.8820010751365675583 ) ) ;
#4591=EDGE_CURVE ( 'NONE', #7650, #9067, #1799, .T. ) ;
#4594=ORIENTED_EDGE ( 'NONE', *, *, #9414, .T. ) ;
#4608=CYLINDRICAL_SURFACE ( 'NONE', #12, 4.000000000000009770 ) ;
#4610=DIRECTION ( 'NONE',  ( 0.000000000000000000, -1.000000000000000000, -0.000000000000000000 ) ) ;
#4617=VECTOR ( 'NONE', #2192, 1000.000000000000000 ) ;
#4620=ADVANCED_FACE ( 'NONE', ( #6641 ), #4817, .F. ) ;
#4629=ORIENTED_EDGE ( 'NONE', *, *, #8880, .T. ) ;
#4653=CIRCLE ( 'NONE', #25, 4.000000000000008882 ) ;
#4654=SHAPE_REPRESENTATION_RELATIONSHIP ( 'NONE' , 'NONE' ,  #5180, #9043 ) ;
#4682=FACE_OUTER_BOUND ( 'NONE', #5941, .T. ) ;
#4703=EDGE_LOOP ( 'NONE', ( #1814, #2615, #4556, #8796, #1561, #10304, #3914, #1140, #8214, #1481, #3950, #8480, #10031, #5978, #3245 ) ) ;
#4707=CIRCLE ( 'NONE', #2061, 4.000000000000008882 ) ;
#4709=AXIS2_PLACEMENT_3D ( 'NONE', #1190, #5977, #8447 ) ;
#4732=ORIENTED_EDGE ( 'NONE', *, *, #5951, .T. ) ;
#4764=SURFACE_SIDE_STYLE ('',( #6204 ) ) ;
#4789=FACE_OUTER_BOUND ( 'NONE', #1308, .T. ) ;
#4808=ORIENTED_EDGE ( 'NONE', *, *, #9552, .F. ) ;
#4817=CYLINDRICAL_SURFACE ( 'NONE', #9183, 4.000000000000009770 ) ;
#4822=ORIENTED_EDGE ( 'NONE', *, *, #670, .T. ) ;
#4824=CARTESIAN_POINT ( 'NONE',  ( -72.90663470096859555, -7.500000000000000000, -371.7168990827444190 ) ) ;
#4837=EDGE_LOOP ( 'NONE', ( #4246, #5068, #2527, #7678 ) ) ;
#4858=VECTOR ( 'NONE', #6300, 1000.000000000000000 ) ;
#4879=FACE_OUTER_BOUND ( 'NONE', #5632, .T. ) ;
#4909=EDGE_CURVE ( 'NONE', #6716, #3828, #1631, .T. ) ;
#4919=LINE ( 'NONE', #3954, #3171 ) ;
#4953=EDGE_CURVE ( 'NONE', #8445, #2874, #912, .T. ) ;
#4961=VERTEX_POINT ( 'NONE', #536 ) ;
#4970=VECTOR ( 'NONE', #968, 1000.000000000000000 ) ;
#4974=DIRECTION ( 'NONE',  ( 0.000000000000000000, -1.000000000000000000, 0.000000000000000000 ) ) ;
#4975=LINE ( 'NONE', #9231, #4541 ) ;
#4992=ORIENTED_EDGE ( 'NONE', *, *, #2791, .T. ) ;
#4995=VECTOR ( 'NONE', #9583, 1000.000000000000000 ) ;
#4996=ORIENTED_EDGE ( 'NONE', *, *, #422, .T. ) ;
#5005=AXIS2_PLACEMENT_3D ( 'NONE', #8670, #2877, #8514 ) ;
#5006=CARTESIAN_POINT ( 'NONE',  ( -85.79375217459825365, -7.500000000000000000, -343.3529193039154279 ) ) ;
#5011=ORIENTED_EDGE ( 'NONE', *, *, #5342, .T. ) ;
#5024=CARTESIAN_POINT ( 'NONE',  ( -101.0297452788102817, -2.500000000000000000, -342.4231267849074811 ) ) ;
#5025=EDGE_LOOP ( 'NONE', ( #750, #2117, #8731, #2917 ) ) ;
#5037=CARTESIAN_POINT ( 'NONE',  ( -86.49427212956700828, -2.500000000000000000, -350.5299153184531633 ) ) ;
#5038=LINE ( 'NONE', #3432, #2669 ) ;
#5044=EDGE_LOOP ( 'NONE', ( #10246, #2862, #8412, #8978, #9696, #9672, #4163, #3434, #390, #354, #1119, #3539, #6964, #10070, #5767 ) ) ;
#5052=ADVANCED_FACE ( 'NONE', ( #1177 ), #4457, .F. ) ;
#5055=DIRECTION ( 'NONE',  ( 0.000000000000000000, -1.000000000000000000, 0.000000000000000000 ) ) ;
#5068=ORIENTED_EDGE ( 'NONE', *, *, #2082, .F. ) ;
#5075=CARTESIAN_POINT ( 'NONE',  ( -80.80421425739181984, -7.500000000000000000, -329.3491872523243842 ) ) ;
#5077=CARTESIAN_POINT ( 'NONE',  ( -46.74071243416547361, -7.500000000000000000, -414.3237589990478114 ) ) ;
#5090=DIRECTION ( 'NONE',  ( -0.8820010751365675583, 0.000000000000000000, -0.4712473909295827323 ) ) ;
#5109=CARTESIAN_POINT ( 'NONE',  ( -79.31727611502927289, -2.500000000000000000, -351.2304352734219606 ) ) ;
#5118=ORIENTED_EDGE ( 'NONE', *, *, #8123, .T. ) ;
#5135=LINE ( 'NONE', #6701, #8630 ) ;
#5143=PLANE ( 'NONE',  #3817 ) ;
#5149=CARTESIAN_POINT ( 'NONE',  ( -102.0103468492230547, -7.500000000000000000, -289.6591388711787545 ) ) ;
#5151=CIRCLE ( 'NONE', #520, 3.499999999999997335 ) ;
#5158=COLOUR_RGB ( '', 0.66274510, 0.83137255, 0.94901961) ;
#5175=EDGE_LOOP ( 'NONE', ( #6756, #1363 ) ) ;
#5180=SHAPE_REPRESENTATION ( 'Handle Mounting Bracket', ( #2817 ), #6445 ) ;
#5188=VERTEX_POINT ( 'NONE', #2573 ) ;
#5210=CARTESIAN_POINT ( 'NONE',  ( -77.77979771402830522, -7.500000000000000000, -385.9384419754180158 ) ) ;
#5221=EDGE_CURVE ( 'NONE', #2124, #8515, #5038, .T. ) ;
#5223=DIRECTION ( 'NONE',  ( 0.000000000000000000, 1.000000000000000000, -0.000000000000000000 ) ) ;
#5227=CIRCLE ( 'NONE', #426, 3.500000000000003997 ) ;
#5234=DIRECTION ( 'NONE',  ( 0.4712473909295827323, 0.000000000000000000, -0.8820010751365675583 ) ) ;
#5246=DIRECTION ( 'NONE',  ( -0.4712473909295827323, 0.000000000000000000, 0.8820010751365675583 ) ) ;
#5247=DIRECTION ( 'NONE',  ( 0.000000000000000000, -1.000000000000000000, 0.000000000000000000 ) ) ;
#5253=EDGE_LOOP ( 'NONE', ( #9350, #257, #4808, #6185 ) ) ;
#5291=ADVANCED_FACE ( 'NONE', ( #789 ), #1751, .F. ) ;
#5299=EDGE_LOOP ( 'NONE', ( #304, #2906, #5118, #1429 ) ) ;
#5308=VECTOR ( 'NONE', #7293, 1000.000000000000000 ) ;
#5320=FACE_OUTER_BOUND ( 'NONE', #5025, .T. ) ;
#5321=DIRECTION ( 'NONE',  ( 0.000000000000000000, 1.000000000000000000, -0.000000000000000000 ) ) ;
#5323=EDGE_LOOP ( 'NONE', ( #1847, #1467, #1152, #3770 ) ) ;
#5342=EDGE_CURVE ( 'NONE', #3089, #8136, #4210, .T. ) ;
#5345=VECTOR ( 'NONE', #3665, 1000.000000000000000 ) ;
#5367=PLANE ( 'NONE',  #316 ) ;
#5383=DIRECTION ( 'NONE',  ( 0.8820010751365675583, 0.000000000000000000, 0.4712473909295827323 ) ) ;
#5387=EDGE_LOOP ( 'NONE', ( #3618, #7032, #3894, #38 ) ) ;
#5390=CYLINDRICAL_SURFACE ( 'NONE', #5005, 14.00000000000000355 ) ;
#5397=LINE ( 'NONE', #1317, #6840 ) ;
#5437=VECTOR ( 'NONE', #7431, 1000.000000000000000 ) ;
#5439=VERTEX_POINT ( 'NONE', #812 ) ;
#5445=CARTESIAN_POINT ( 'NONE',  ( -102.0103468492230547, -2.500000000000000000, -289.6591388711787545 ) ) ;
#5448=VECTOR ( 'NONE', #7026, 1000.000000000000000 ) ;
#5461=ORIENTED_EDGE ( 'NONE', *, *, #7790, .T. ) ;
#5464=CYLINDRICAL_SURFACE ( 'NONE', #7765, 5.000000000000006217 ) ;
#5472=VECTOR ( 'NONE', #2996, 1000.000000000000000 ) ;
#5476=CARTESIAN_POINT ( 'NONE',  ( -100.2082379103963063, -7.500000000000000000, -339.7166298527751565 ) ) ;
#5492=AXIS2_PLACEMENT_3D ( 'NONE', #3285, #5055, #3451 ) ;
#5543=CARTESIAN_POINT ( 'NONE',  ( -72.90663470096859555, -2.500000000000000000, -371.7168990827444190 ) ) ;
#5548=VERTEX_POINT ( 'NONE', #120 ) ;
#5553=EDGE_CURVE ( 'NONE', #6664, #6471, #7686, .T. ) ;
#5554=CLOSED_SHELL ( 'NONE', ( #6120, #9252, #3446, #7191, #9502, #3121, #7268, #1485, #3589, #4308, #3189, #3113, #3818, #9892, #7391, #1477, #3669, #6945, #5664, #6727, #3658, #4620, #1535, #5052, #9969, #10611, #1943, #5291, #2575 ) ) ;
#5562=ORIENTED_EDGE ( 'NONE', *, *, #9616, .F. ) ;
#5585=CARTESIAN_POINT ( 'NONE',  ( -46.74071243416547361, -2.500000000000000000, -414.3237589990478114 ) ) ;
#5625=DIRECTION ( 'NONE',  ( -0.9968876850330226080, 0.000000000000000000, 0.07883491250392142546 ) ) ;
#5629=PLANE ( 'NONE',  #5709 ) ;
#5632=EDGE_LOOP ( 'NONE', ( #1257, #6461, #4996, #3563 ) ) ;
#5664=ADVANCED_FACE ( 'NONE', ( #7950 ), #1286, .T. ) ;
#5672=ORIENTED_EDGE ( 'NONE', *, *, #7837, .T. ) ;
#5689=CIRCLE ( 'NONE', #6907, 1.999999999999998224 ) ;
#5697=CIRCLE ( 'NONE', #8073, 4.000000000000008882 ) ;
#5700=FILL_AREA_STYLE ('',( #7426 ) ) ;
#5703=DIRECTION ( 'NONE',  ( 0.000000000000000000, -1.000000000000000000, 0.000000000000000000 ) ) ;
#5709=AXIS2_PLACEMENT_3D ( 'NONE', #6769, #9934, #1874 ) ;
#5739=VERTEX_POINT ( 'NONE', #7149 ) ;
#5748=DIRECTION ( 'NONE',  ( 0.000000000000000000, -1.000000000000000000, 0.000000000000000000 ) ) ;
#5752=EDGE_CURVE ( 'NONE', #8575, #5439, #6731, .T. ) ;
#5755=ORIENTED_EDGE ( 'NONE', *, *, #7155, .F. ) ;
#5758=CARTESIAN_POINT ( 'NONE',  ( -98.44423576012317767, -7.500000000000000000, -338.7741350709160315 ) ) ;
#5762=ORIENTED_EDGE ( 'NONE', *, *, #10192, .F. ) ;
#5767=ORIENTED_EDGE ( 'NONE', *, *, #1774, .T. ) ;
#5773=EDGE_LOOP ( 'NONE', ( #8949, #1432 ) ) ;
#5789=ORIENTED_EDGE ( 'NONE', *, *, #568, .F. ) ;
#5794=AXIS2_PLACEMENT_3D ( 'NONE', #1344, #2261, #7154 ) ;
#5799=ORIENTED_EDGE ( 'NONE', *, *, #1869, .T. ) ;
#5803=CARTESIAN_POINT ( 'NONE',  ( -99.26574312853713877, -2.500000000000000000, -341.4806320030483562 ) ) ;
#5809=DIRECTION ( 'NONE',  ( -0.8820010751365653379, 0.000000000000000000, -0.4712473909295871732 ) ) ;
#5826=EDGE_LOOP ( 'NONE', ( #4193, #4534 ) ) ;
#5835=EDGE_CURVE ( 'NONE', #1301, #4961, #3170, .T. ) ;
#5886=DIRECTION ( 'NONE',  ( 0.000000000000000000, -1.000000000000000000, 0.000000000000000000 ) ) ;
#5902=CIRCLE ( 'NONE', #1266, 13.99999999999999645 ) ;
#5917=AXIS2_PLACEMENT_3D ( 'NONE', #6042, #1915, #3681 ) ;
#5925=CARTESIAN_POINT ( 'NONE',  ( -98.44423576012317767, -2.500000000000000000, -338.7741350709160315 ) ) ;
#5927=VERTEX_POINT ( 'NONE', #5149 ) ;
#5941=EDGE_LOOP ( 'NONE', ( #3021, #6810, #6910, #3297 ) ) ;
#5951=EDGE_CURVE ( 'NONE', #3089, #5548, #9081, .T. ) ;
#5970=AXIS2_PLACEMENT_3D ( 'NONE', #2103, #7956, #9463 ) ;
#5977=DIRECTION ( 'NONE',  ( 0.4712473909295827323, 0.000000000000000000, -0.8820010751365675583 ) ) ;
#5978=ORIENTED_EDGE ( 'NONE', *, *, #5221, .T. ) ;
#5984=CARTESIAN_POINT ( 'NONE',  ( -119.6503683519543983, -7.500000000000000000, -299.0840866897705155 ) ) ;
#5999=DIRECTION ( 'NONE',  ( -0.8820010751365675583, 0.000000000000000000, -0.4712473909295827323 ) ) ;
#6005=DIRECTION ( 'NONE',  ( 0.000000000000000000, -1.000000000000000000, 0.000000000000000000 ) ) ;
#6007=EDGE_CURVE ( 'NONE', #2874, #320, #5689, .T. ) ;
#6012=CARTESIAN_POINT ( 'NONE',  ( -86.49427212956700828, -7.500000000000000000, -350.5299153184531633 ) ) ;
#6023=( GEOMETRIC_REPRESENTATION_CONTEXT ( 3 ) GLOBAL_UNCERTAINTY_ASSIGNED_CONTEXT ( ( #6354 ) ) GLOBAL_UNIT_ASSIGNED_CONTEXT ( ( #713, #1625, #4206 ) ) REPRESENTATION_CONTEXT ( 'NONE', 'WORKASPACE' ) );
#6042=CARTESIAN_POINT ( 'NONE',  ( -46.74071243416547361, -2.500000000000000000, -414.3237589990478114 ) ) ;
#6047=CARTESIAN_POINT ( 'NONE',  ( -119.6503683519543983, -2.500000000000000000, -299.0840866897705155 ) ) ;
#6075=CARTESIAN_POINT ( 'NONE',  ( -80.80421425739181984, -2.500000000000000000, -329.3491872523243842 ) ) ;
#6087=ORIENTED_EDGE ( 'NONE', *, *, #2998, .T. ) ;
#6088=VECTOR ( 'NONE', #889, 1000.000000000000000 ) ;
#6095=ORIENTED_EDGE ( 'NONE', *, *, #670, .F. ) ;
#6096=COLOUR_RGB ( '', 0.66274510, 0.83137255, 0.94901961) ;
#6116=FACE_OUTER_BOUND ( 'NONE', #6745, .T. ) ;
#6120=ADVANCED_FACE ( 'NONE', ( #9335 ), #5390, .T. ) ;
#6124=CARTESIAN_POINT ( 'NONE',  ( -86.49427212956700828, -2.500000000000000000, -350.5299153184531633 ) ) ;
#6140=CYLINDRICAL_SURFACE ( 'NONE', #9632, 3.499999999999997335 ) ;
#6151=EDGE_CURVE ( 'NONE', #4003, #8834, #2267, .T. ) ;
#6154=CARTESIAN_POINT ( 'NONE',  ( -85.79375217459825365, -2.500000000000000000, -343.3529193039154279 ) ) ;
#6163=EDGE_CURVE ( 'NONE', #7707, #269, #1755, .T. ) ;
#6174=CARTESIAN_POINT ( 'NONE',  ( -84.02975002432511076, -7.500000000000000000, -342.4104245220563030 ) ) ;
#6183=LINE ( 'NONE', #7799, #6887 ) ;
#6185=ORIENTED_EDGE ( 'NONE', *, *, #7641, .F. ) ;
#6196=ORIENTED_EDGE ( 'NONE', *, *, #363, .T. ) ;
#6204=SURFACE_STYLE_FILL_AREA ( #2077 ) ;
#6205=EDGE_CURVE ( 'NONE', #56, #3871, #10341, .T. ) ;
#6232=AXIS2_PLACEMENT_3D ( 'NONE', #2302, #4610, #3916 ) ;
#6238=DIRECTION ( 'NONE',  ( 0.8820010751365678914, 0.000000000000000000, 0.4712473909295818442 ) ) ;
#6245=CARTESIAN_POINT ( 'NONE',  ( -46.74071243416547361, -7.500000000000000000, -414.3237589990478114 ) ) ;
#6264=CARTESIAN_POINT ( 'NONE',  ( -81.08127826530241578, -2.500000000000000000, -352.1729300552810855 ) ) ;
#6286=DIRECTION ( 'NONE',  ( 0.000000000000000000, 1.000000000000000000, -0.000000000000000000 ) ) ;
#6300=DIRECTION ( 'NONE',  ( 0.8820010751365675583, 0.000000000000000000, 0.4712473909295827323 ) ) ;
#6337=DIRECTION ( 'NONE',  ( -0.4712473909295827323, 0.000000000000000000, 0.8820010751365675583 ) ) ;
#6354=UNCERTAINTY_MEASURE_WITH_UNIT (LENGTH_MEASURE( 1.000000000000000082E-05 ), #713, 'distance_accuracy_value', 'NONE');
#6360=EDGE_LOOP ( 'NONE', ( #7465, #6095, #5672, #1170 ) ) ;
#6378=VECTOR ( 'NONE', #216, 1000.000000000000000 ) ;
#6385=CARTESIAN_POINT ( 'NONE',  ( -101.9722400606694350, -2.500000000000000000, -340.6591246346343382 ) ) ;
#6411=LINE ( 'NONE', #3193, #4858 ) ;
#6419=CARTESIAN_POINT ( 'NONE',  ( -82.96626782902075092, -7.500000000000000000, -348.6449257547347997 ) ) ;
#6444=CARTESIAN_POINT ( 'NONE',  ( -86.49427212956700828, -2.500000000000000000, -350.5299153184531633 ) ) ;
#6445=( GEOMETRIC_REPRESENTATION_CONTEXT ( 3 ) GLOBAL_UNCERTAINTY_ASSIGNED_CONTEXT ( ( #1950 ) ) GLOBAL_UNIT_ASSIGNED_CONTEXT ( ( #10396, #9593, #8618 ) ) REPRESENTATION_CONTEXT ( 'NONE', 'WORKASPACE' ) );
#6447=DIRECTION ( 'NONE',  ( 0.000000000000000000, -1.000000000000000000, 0.000000000000000000 ) ) ;
#6449=PRODUCT_DEFINITION_FORMATION_WITH_SPECIFIED_SOURCE ( 'ANY', '', #8784, .NOT_KNOWN. ) ;
#6461=ORIENTED_EDGE ( 'NONE', *, *, #7066, .T. ) ;
#6465=FACE_OUTER_BOUND ( 'NONE', #9587, .T. ) ;
#6471=VERTEX_POINT ( 'NONE', #290 ) ;
#6475=DIRECTION ( 'NONE',  ( 0.000000000000000000, -1.000000000000000000, 0.000000000000000000 ) ) ;
#6531=AXIS2_PLACEMENT_3D ( 'NONE', #636, #4018, #5625 ) ;
#6557=FACE_OUTER_BOUND ( 'NONE', #5044, .T. ) ;
#6564=DIRECTION ( 'NONE',  ( 0.000000000000000000, 1.000000000000000000, -0.000000000000000000 ) ) ;
#6584=DIRECTION ( 'NONE',  ( -0.9968876850330226080, 0.000000000000000000, 0.07883491250392142546 ) ) ;
#6592=VECTOR ( 'NONE', #3899, 1000.000000000000000 ) ;
#6600=EDGE_CURVE ( 'NONE', #7778, #9710, #9322, .T. ) ;
#6602=DIRECTION ( 'NONE',  ( 0.4712473909295827323, 0.000000000000000000, -0.8820010751365675583 ) ) ;
#6620=CARTESIAN_POINT ( 'NONE',  ( -91.84750071659622961, -7.500000000000000000, -370.2190357451694922 ) ) ;
#6640=EDGE_CURVE ( 'NONE', #1418, #6862, #5697, .T. ) ;
#6641=FACE_OUTER_BOUND ( 'NONE', #3247, .T. ) ;
#6645=EDGE_LOOP ( 'NONE', ( #8327, #8993, #3276, #9281 ) ) ;
#6647=FACE_OUTER_BOUND ( 'NONE', #3474, .T. ) ;
#6664=VERTEX_POINT ( 'NONE', #9422 ) ;
#6688=VECTOR ( 'NONE', #5748, 1000.000000000000000 ) ;
#6701=CARTESIAN_POINT ( 'NONE',  ( -87.43676691142619006, -2.500000000000000000, -348.7659131681800773 ) ) ;
#6713=EDGE_CURVE ( 'NONE', #8834, #4003, #2064, .T. ) ;
#6716=VERTEX_POINT ( 'NONE', #66 ) ;
#6727=ADVANCED_FACE ( 'NONE', ( #7531 ), #8280, .F. ) ;
#6731=CIRCLE ( 'NONE', #7583, 1.999999999999980238 ) ;
#6741=AXIS2_PLACEMENT_3D ( 'NONE', #4293, #5999, #4240 ) ;
#6745=EDGE_LOOP ( 'NONE', ( #8930, #10342, #1493, #2177 ) ) ;
#6755=CARTESIAN_POINT ( 'NONE',  ( -100.2082379103963063, -7.500000000000000000, -339.7166298527751565 ) ) ;
#6756=ORIENTED_EDGE ( 'NONE', *, *, #8507, .T. ) ;
#6758=CARTESIAN_POINT ( 'NONE',  ( -82.18980308971114823, -2.366295999999999733, -388.2946789300659134 ) ) ;
#6769=CARTESIAN_POINT ( 'NONE',  ( -77.27620995684556249, -2.500000000000000000, -327.4641976886060206 ) ) ;
#6781=VECTOR ( 'NONE', #4590, 1000.000000000000000 ) ;
#6782=VECTOR ( 'NONE', #2588, 1000.000000000000000 ) ;
#6810=ORIENTED_EDGE ( 'NONE', *, *, #8293, .T. ) ;
#6824=EDGE_CURVE ( 'NONE', #8080, #3828, #10060, .T. ) ;
#6835=DIRECTION ( 'NONE',  ( 0.4712473909295827323, 0.000000000000000000, -0.8820010751365675583 ) ) ;
#6840=VECTOR ( 'NONE', #5246, 1000.000000000000000 ) ;
#6844=CARTESIAN_POINT ( 'NONE',  ( -69.81963093799060971, -2.500000000000000000, -370.0675332144908793 ) ) ;
#6846=CARTESIAN_POINT ( 'NONE',  ( -119.6503683519543983, -2.500000000000000000, -299.0840866897705155 ) ) ;
#6851=ORIENTED_EDGE ( 'NONE', *, *, #2921, .T. ) ;
#6856=CARTESIAN_POINT ( 'NONE',  ( -85.25464975288055314, -2.500000000000000000, -378.3143625557585779 ) ) ;
#6862=VERTEX_POINT ( 'NONE', #476 ) ;
#6870=LINE ( 'NONE', #8617, #5448 ) ;
#6884=AXIS2_PLACEMENT_3D ( 'NONE', #1607, #7243, #10514 ) ;
#6887=VECTOR ( 'NONE', #1351, 1000.000000000000000 ) ;
#6907=AXIS2_PLACEMENT_3D ( 'NONE', #1718, #6005, #1011 ) ;
#6910=ORIENTED_EDGE ( 'NONE', *, *, #5553, .F. ) ;
#6930=EDGE_CURVE ( 'NONE', #2607, #6716, #230, .T. ) ;
#6936=DIRECTION ( 'NONE',  ( 0.8820010751365678914, 0.000000000000000000, 0.4712473909295818442 ) ) ;
#6945=ADVANCED_FACE ( 'NONE', ( #1327 ), #4608, .F. ) ;
#6957=CARTESIAN_POINT ( 'NONE',  ( -82.14476046060677561, -7.500000000000000000, -345.9384288226025888 ) ) ;
#6964=ORIENTED_EDGE ( 'NONE', *, *, #2731, .T. ) ;
#6973=CARTESIAN_POINT ( 'NONE',  ( -75.99363846394659561, -2.500000000000000000, -373.3662649509979587 ) ) ;
#6982=ORIENTED_EDGE ( 'NONE', *, *, #7327, .T. ) ;
#6987=DIRECTION ( 'NONE',  ( 0.000000000000000000, 1.000000000000000000, -0.000000000000000000 ) ) ;
#6998=ORIENTED_EDGE ( 'NONE', *, *, #4953, .F. ) ;
#7026=DIRECTION ( 'NONE',  ( 0.000000000000000000, 1.000000000000000000, -0.000000000000000000 ) ) ;
#7027=( NAMED_UNIT ( * ) SI_UNIT ( $, .STERADIAN. ) SOLID_ANGLE_UNIT ( ) );
#7032=ORIENTED_EDGE ( 'NONE', *, *, #3893, .F. ) ;
#7039=CARTESIAN_POINT ( 'NONE',  ( -75.99363846394659561, -7.500000000000000000, -373.3662649509979587 ) ) ;
#7053=AXIS2_PLACEMENT_3D ( 'NONE', #5803, #6564, #65 ) ;
#7063=EDGE_LOOP ( 'NONE', ( #6998, #5762, #6087, #8084 ) ) ;
#7066=EDGE_CURVE ( 'NONE', #8626, #306, #529, .T. ) ;
#7080=ORIENTED_EDGE ( 'NONE', *, *, #977, .F. ) ;
#7104=DIRECTION ( 'NONE',  ( 0.000000000000000000, 1.000000000000000000, -0.000000000000000000 ) ) ;
#7123=EDGE_LOOP ( 'NONE', ( #10605, #4403, #5799, #4282 ) ) ;
#7149=CARTESIAN_POINT ( 'NONE',  ( -100.2082379103963063, -2.500000000000000000, -339.7166298527751565 ) ) ;
#7154=DIRECTION ( 'NONE',  ( 0.4712473909295827323, 0.000000000000000000, -0.8820010751365675583 ) ) ;
#7155=EDGE_CURVE ( 'NONE', #10171, #7605, #2222, .T. ) ;
#7191=ADVANCED_FACE ( 'NONE', ( #4879 ), #8157, .T. ) ;
#7206=EDGE_CURVE ( 'NONE', #5548, #3094, #3375, .T. ) ;
#7207=FACE_BOUND ( 'NONE', #5773, .T. ) ;
#7211=DIRECTION ( 'NONE',  ( 0.000000000000000000, -1.000000000000000000, 0.000000000000000000 ) ) ;
#7215=CARTESIAN_POINT ( 'NONE',  ( -72.90663470096859555, -7.500000000000000000, -371.7168990827444190 ) ) ;
#7233=LINE ( 'NONE', #9810, #6592 ) ;
#7243=DIRECTION ( 'NONE',  ( 0.000000000000000000, 1.000000000000000000, -0.000000000000000000 ) ) ;
#7258=CYLINDRICAL_SURFACE ( 'NONE', #7456, 4.000000000000008882 ) ;
#7268=ADVANCED_FACE ( 'NONE', ( #3318 ), #895, .T. ) ;
#7282=CARTESIAN_POINT ( 'NONE',  ( -46.74071243416547361, -2.500000000000000000, -414.3237589990478114 ) ) ;
#7293=DIRECTION ( 'NONE',  ( 0.000000000000000000, -1.000000000000000000, 0.000000000000000000 ) ) ;
#7296=DIRECTION ( 'NONE',  ( 0.000000000000000000, 1.000000000000000000, -0.000000000000000000 ) ) ;
#7305=CARTESIAN_POINT ( 'NONE',  ( -79.04021210711869116, -2.500000000000000000, -328.4066924704651456 ) ) ;
#7327=EDGE_CURVE ( 'NONE', #8080, #8626, #7710, .T. ) ;
#7340=DIRECTION ( 'NONE',  ( 0.000000000000000000, 1.000000000000000000, -0.000000000000000000 ) ) ;
#7341=AXIS2_PLACEMENT_3D ( 'NONE', #8647, #4572, #7846 ) ;
#7356=DIRECTION ( 'NONE',  ( -0.8820010751365675583, 0.000000000000000000, -0.4712473909295827323 ) ) ;
#7359=DIRECTION ( 'NONE',  ( 0.4712473909295827323, 0.000000000000000000, -0.8820010751365675583 ) ) ;
#7383=DIRECTION ( 'NONE',  ( -0.8820010751365716661, 0.000000000000000000, -0.4712473909295749053 ) ) ;
#7391=ADVANCED_FACE ( 'NONE', ( #6465 ), #1685, .T. ) ;
#7392=DIRECTION ( 'NONE',  ( 0.000000000000000000, 1.000000000000000000, -0.000000000000000000 ) ) ;
#7397=ORIENTED_EDGE ( 'NONE', *, *, #2353, .T. ) ;
#7407=DIRECTION ( 'NONE',  ( 0.000000000000000000, -1.000000000000000000, 0.000000000000000000 ) ) ;
#7426=FILL_AREA_STYLE_COLOUR ( '', #5158 ) ;
#7431=DIRECTION ( 'NONE',  ( 0.000000000000000000, -1.000000000000000000, 0.000000000000000000 ) ) ;
#7443=APPLICATION_CONTEXT ( 'automotive_design' ) ;
#7448=DIRECTION ( 'NONE',  ( 0.8820010751365653379, 0.000000000000000000, 0.4712473909295871732 ) ) ;
#7452=LINE ( 'NONE', #1757, #2644 ) ;
#7456=AXIS2_PLACEMENT_3D ( 'NONE', #8058, #6447, #703 ) ;
#7465=ORIENTED_EDGE ( 'NONE', *, *, #5221, .F. ) ;
#7478=CARTESIAN_POINT ( 'NONE',  ( -101.0297452788102817, -2.500000000000000000, -342.4231267849074811 ) ) ;
#7480=LINE ( 'NONE', #10593, #10148 ) ;
#7531=FACE_OUTER_BOUND ( 'NONE', #6645, .T. ) ;
#7537=CARTESIAN_POINT ( 'NONE',  ( -77.77979771402830522, -2.500000000000000000, -385.9384419754180158 ) ) ;
#7546=AXIS2_PLACEMENT_3D ( 'NONE', #4234, #9180, #1818 ) ;
#7553=DIRECTION ( 'NONE',  ( -0.8820010751365675583, 0.000000000000000000, -0.4712473909295827323 ) ) ;
#7563=VERTEX_POINT ( 'NONE', #9856 ) ;
#7579=DIRECTION ( 'NONE',  ( -0.8820010751365678914, 0.000000000000000000, -0.4712473909295818442 ) ) ;
#7583=AXIS2_PLACEMENT_3D ( 'NONE', #10417, #3059, #8805 ) ;
#7589=DIRECTION ( 'NONE',  ( 0.000000000000000000, -1.000000000000000000, 0.000000000000000000 ) ) ;
#7605=VERTEX_POINT ( 'NONE', #5006 ) ;
#7617=VECTOR ( 'NONE', #6475, 1000.000000000000000 ) ;
#7641=EDGE_CURVE ( 'NONE', #1301, #3871, #9781, .T. ) ;
#7650=VERTEX_POINT ( 'NONE', #8393 ) ;
#7666=LINE ( 'NONE', #8613, #581 ) ;
#7667=CARTESIAN_POINT ( 'NONE',  ( -46.74071243416547361, -7.500000000000000000, -414.3237589990478114 ) ) ;
#7678=ORIENTED_EDGE ( 'NONE', *, *, #9552, .T. ) ;
#7686=LINE ( 'NONE', #5210, #8957 ) ;
#7689=AXIS2_PLACEMENT_3D ( 'NONE', #7831, #10208, #10151 ) ;
#7707=VERTEX_POINT ( 'NONE', #6844 ) ;
#7710=CIRCLE ( 'NONE', #9275, 14.00000000000000888 ) ;
#7732=CARTESIAN_POINT ( 'NONE',  ( -69.81963093799060971, -7.500000000000000000, -370.0675332144908793 ) ) ;
#7765=AXIS2_PLACEMENT_3D ( 'NONE', #3002, #8687, #8579 ) ;
#7778=VERTEX_POINT ( 'NONE', #7537 ) ;
#7784=DIRECTION ( 'NONE',  ( 0.000000000000000000, 1.000000000000000000, -0.000000000000000000 ) ) ;
#7790=EDGE_CURVE ( 'NONE', #1052, #1373, #9033, .T. ) ;
#7799=CARTESIAN_POINT ( 'NONE',  ( -79.31727611502927289, -7.500000000000000000, -351.2304352734219606 ) ) ;
#7801=ORIENTED_EDGE ( 'NONE', *, *, #3927, .F. ) ;
#7827=LINE ( 'NONE', #8576, #9007 ) ;
#7830=EDGE_CURVE ( 'NONE', #8136, #1418, #9623, .T. ) ;
#7831=CARTESIAN_POINT ( 'NONE',  ( -91.84750071659622961, -2.500000000000000000, -370.2190357451694922 ) ) ;
#7837=EDGE_CURVE ( 'NONE', #1738, #5739, #2479, .T. ) ;
#7846=DIRECTION ( 'NONE',  ( 0.4712473909295803454, 0.000000000000000000, -0.8820010751365688906 ) ) ;
#7855=CARTESIAN_POINT ( 'NONE',  ( -98.44423576012317767, -2.500000000000000000, -338.7741350709160315 ) ) ;
#7865=ORIENTED_EDGE ( 'NONE', *, *, #3893, .T. ) ;
#7879=EDGE_LOOP ( 'NONE', ( #9526, #8973, #5562, #6196 ) ) ;
#7918=ORIENTED_EDGE ( 'NONE', *, *, #7924, .F. ) ;
#7924=EDGE_CURVE ( 'NONE', #2607, #9600, #4305, .T. ) ;
#7950=FACE_OUTER_BOUND ( 'NONE', #4837, .T. ) ;
#7956=DIRECTION ( 'NONE',  ( 0.8820010751365675583, 0.000000000000000000, 0.4712473909295827323 ) ) ;
#7969=AXIS2_PLACEMENT_3D ( 'NONE', #9509, #7784, #9456 ) ;
#7977=EDGE_CURVE ( 'NONE', #4961, #10171, #2694, .T. ) ;
#7979=VECTOR ( 'NONE', #7986, 1000.000000000000000 ) ;
#7986=DIRECTION ( 'NONE',  ( -0.4712473909295827323, 0.000000000000000000, 0.8820010751365675583 ) ) ;
#7998=DIRECTION ( 'NONE',  ( -0.8820010751365653379, 0.000000000000000000, -0.4712473909295871732 ) ) ;
#8024=CARTESIAN_POINT ( 'NONE',  ( -34.39269738225353024, -2.500000000000000000, -407.7262955260336525 ) ) ;
#8028=ORIENTED_EDGE ( 'NONE', *, *, #6713, .T. ) ;
#8052=DIRECTION ( 'NONE',  ( -0.8820010751365675583, 0.000000000000000000, -0.4712473909295827323 ) ) ;
#8055=VECTOR ( 'NONE', #7211, 1000.000000000000000 ) ;
#8056=CIRCLE ( 'NONE', #512, 4.999999999999985789 ) ;
#8058=CARTESIAN_POINT ( 'NONE',  ( -83.90876261087991850, -2.366295999999999733, -346.8809236044617137 ) ) ;
#8073=AXIS2_PLACEMENT_3D ( 'NONE', #6957, #10231, #2865 ) ;
#8074=LINE ( 'NONE', #9741, #9782 ) ;
#8078=CARTESIAN_POINT ( 'NONE',  ( -99.26574312853713877, -7.656480000000000175, -341.4806320030483562 ) ) ;
#8080=VERTEX_POINT ( 'NONE', #9453 ) ;
#8084=ORIENTED_EDGE ( 'NONE', *, *, #8123, .F. ) ;
#8104=LINE ( 'NONE', #7305, #10460 ) ;
#8116=SHAPE_DEFINITION_REPRESENTATION ( #10419, #5180 ) ;
#8123=EDGE_CURVE ( 'NONE', #2874, #5439, #1126, .T. ) ;
#8136=VERTEX_POINT ( 'NONE', #425 ) ;
#8157=CYLINDRICAL_SURFACE ( 'NONE', #3940, 14.00000000000000355 ) ;
#8170=DIRECTION ( 'NONE',  ( -0.8820010751365675583, 0.000000000000000000, -0.4712473909295827323 ) ) ;
#8175=EDGE_CURVE ( 'NONE', #8575, #1218, #8104, .T. ) ;
#8189=EDGE_LOOP ( 'NONE', ( #394, #2671, #2940, #473, #10559, #2497, #9808, #3695 ) ) ;
#8195=DIRECTION ( 'NONE',  ( -0.9968876850330226080, 0.000000000000000000, 0.07883491250392142546 ) ) ;
#8202=VERTEX_POINT ( 'NONE', #4078 ) ;
#8214=ORIENTED_EDGE ( 'NONE', *, *, #6007, .T. ) ;
#8251=CARTESIAN_POINT ( 'NONE',  ( -80.80421425739181984, -2.500000000000000000, -329.3491872523243842 ) ) ;
#8259=MECHANICAL_DESIGN_GEOMETRIC_PRESENTATION_REPRESENTATION('',(#531),#6023);
#8261=PLANE ( 'NONE',  #6741 ) ;
#8270=AXIS2_PLACEMENT_3D ( 'NONE', #7282, #8890, #10558 ) ;
#8280=CYLINDRICAL_SURFACE ( 'NONE', #5492, 4.000000000000008882 ) ;
#8293=EDGE_CURVE ( 'NONE', #9710, #6471, #2350, .T. ) ;
#8304=LINE ( 'NONE', #8251, #6088 ) ;
#8327=ORIENTED_EDGE ( 'NONE', *, *, #2082, .T. ) ;
#8333=CARTESIAN_POINT ( 'NONE',  ( -72.90663470096859555, -2.500000000000000000, -371.7168990827444190 ) ) ;
#8346=DIRECTION ( 'NONE',  ( -0.8820010751365675583, 0.000000000000000000, -0.4712473909295827323 ) ) ;
#8355=DIRECTION ( 'NONE',  ( 0.000000000000000000, 1.000000000000000000, -0.000000000000000000 ) ) ;
#8393=CARTESIAN_POINT ( 'NONE',  ( -85.25464975288055314, -7.500000000000000000, -378.3143625557585779 ) ) ;
#8400=ORIENTED_EDGE ( 'NONE', *, *, #1881, .T. ) ;
#8412=ORIENTED_EDGE ( 'NONE', *, *, #10296, .F. ) ;
#8419=FACE_OUTER_BOUND ( 'NONE', #509, .T. ) ;
#8445=VERTEX_POINT ( 'NONE', #1749 ) ;
#8447=DIRECTION ( 'NONE',  ( -0.8820010751365675583, 0.000000000000000000, -0.4712473909295827323 ) ) ;
#8474=ORIENTED_EDGE ( 'NONE', *, *, #7830, .F. ) ;
#8480=ORIENTED_EDGE ( 'NONE', *, *, #10150, .T. ) ;
#8484=AXIS2_PLACEMENT_3D ( 'NONE', #1034, #5223, #241 ) ;
#8507=EDGE_CURVE ( 'NONE', #932, #5188, #5151, .T. ) ;
#8513=ORIENTED_EDGE ( 'NONE', *, *, #10192, .T. ) ;
#8514=DIRECTION ( 'NONE',  ( -0.8820010751365676693, 0.000000000000000000, -0.4712473909295822883 ) ) ;
#8515=VERTEX_POINT ( 'NONE', #6755 ) ;
#8516=DIRECTION ( 'NONE',  ( 0.8820010751365664481, 0.000000000000000000, 0.4712473909295847307 ) ) ;
#8531=VECTOR ( 'NONE', #6987, 1000.000000000000000 ) ;
#8561=VERTEX_POINT ( 'NONE', #5075 ) ;
#8575=VERTEX_POINT ( 'NONE', #3017 ) ;
#8576=CARTESIAN_POINT ( 'NONE',  ( -43.65370867118748777, -7.500000000000000000, -412.6743931307942717 ) ) ;
#8579=DIRECTION ( 'NONE',  ( 0.9968876850330226080, 0.000000000000000000, -0.07883491250392217486 ) ) ;
#8604=CARTESIAN_POINT ( 'NONE',  ( -85.79375217459825365, -2.500000000000000000, -343.3529193039154279 ) ) ;
#8613=CARTESIAN_POINT ( 'NONE',  ( -77.77979771402830522, -2.500000000000000000, -385.9384419754180158 ) ) ;
#8617=CARTESIAN_POINT ( 'NONE',  ( -79.04021210711869116, -7.500000000000000000, -328.4066924704651456 ) ) ;
#8618=( NAMED_UNIT ( * ) SI_UNIT ( $, .STERADIAN. ) SOLID_ANGLE_UNIT ( ) );
#8626=VERTEX_POINT ( 'NONE', #6856 ) ;
#8630=VECTOR ( 'NONE', #948, 1000.000000000000000 ) ;
#8634=CARTESIAN_POINT ( 'NONE',  ( 0.000000000000000000, 0.000000000000000000, 0.000000000000000000 ) ) ;
#8646=ORIENTED_EDGE ( 'NONE', *, *, #2698, .F. ) ;
#8647=CARTESIAN_POINT ( 'NONE',  ( -81.20226567874760804, -2.500000000000000000, -347.7024309728756748 ) ) ;
#8670=CARTESIAN_POINT ( 'NONE',  ( -72.90663470096859555, -2.500000000000000000, -371.7168990827444190 ) ) ;
#8676=PRESENTATION_STYLE_ASSIGNMENT (( #10349 ) ) ;
#8685=CARTESIAN_POINT ( 'NONE',  ( -101.0297452788102817, -7.500000000000000000, -342.4231267849074811 ) ) ;
#8687=DIRECTION ( 'NONE',  ( 0.000000000000000000, -1.000000000000000000, 0.000000000000000000 ) ) ;
#8692=DIRECTION ( 'NONE',  ( -0.4712473909295827323, 0.000000000000000000, 0.8820010751365675583 ) ) ;
#8706=VECTOR ( 'NONE', #3805, 1000.000000000000000 ) ;
#8731=ORIENTED_EDGE ( 'NONE', *, *, #2712, .T. ) ;
#8740=EDGE_LOOP ( 'NONE', ( #4594, #10495 ) ) ;
#8757=DIRECTION ( 'NONE',  ( 0.000000000000000000, -1.000000000000000000, 0.000000000000000000 ) ) ;
#8776=DIRECTION ( 'NONE',  ( 0.8820010751365678914, 0.000000000000000000, 0.4712473909295818442 ) ) ;
#8780=DIRECTION ( 'NONE',  ( 0.000000000000000000, -1.000000000000000000, 0.000000000000000000 ) ) ;
#8784=PRODUCT ( 'Handle Mounting Bracket', 'Handle Mounting Bracket', '', ( #1460 ) ) ;
#8796=ORIENTED_EDGE ( 'NONE', *, *, #4591, .T. ) ;
#8798=FACE_BOUND ( 'NONE', #8740, .T. ) ;
#8805=DIRECTION ( 'NONE',  ( -0.4712473909295860630, 0.000000000000000000, 0.8820010751365656709 ) ) ;
#8834=VERTEX_POINT ( 'NONE', #4042 ) ;
#8844=( GEOMETRIC_REPRESENTATION_CONTEXT ( 3 ) GLOBAL_UNCERTAINTY_ASSIGNED_CONTEXT ( ( #9153 ) ) GLOBAL_UNIT_ASSIGNED_CONTEXT ( ( #465, #3091, #7027 ) ) REPRESENTATION_CONTEXT ( 'NONE', 'WORKASPACE' ) );
#8866=DIRECTION ( 'NONE',  ( 0.000000000000000000, -1.000000000000000000, 0.000000000000000000 ) ) ;
#8877=ORIENTED_EDGE ( 'NONE', *, *, #4382, .F. ) ;
#8880=EDGE_CURVE ( 'NONE', #9600, #700, #9143, .T. ) ;
#8883=CIRCLE ( 'NONE', #9567, 1.999999999999980238 ) ;
#8884=DIRECTION ( 'NONE',  ( -0.9968876850330226080, 0.000000000000000000, 0.07883491250392142546 ) ) ;
#8887=ORIENTED_EDGE ( 'NONE', *, *, #10397, .F. ) ;
#8890=DIRECTION ( 'NONE',  ( 0.000000000000000000, 1.000000000000000000, -0.000000000000000000 ) ) ;
#8908=EDGE_CURVE ( 'NONE', #269, #7707, #251, .T. ) ;
#8928=DIRECTION ( 'NONE',  ( -0.4712473909295803454, 0.000000000000000000, 0.8820010751365688906 ) ) ;
#8930=ORIENTED_EDGE ( 'NONE', *, *, #6824, .T. ) ;
#8933=DIRECTION ( 'NONE',  ( 0.000000000000000000, -1.000000000000000000, 0.000000000000000000 ) ) ;
#8949=ORIENTED_EDGE ( 'NONE', *, *, #8908, .F. ) ;
#8952=CARTESIAN_POINT ( 'NONE',  ( -59.08872748607741698, -2.500000000000000000, -420.9212224720619702 ) ) ;
#8957=VECTOR ( 'NONE', #10004, 1000.000000000000000 ) ;
#8973=ORIENTED_EDGE ( 'NONE', *, *, #10074, .F. ) ;
#8975=ORIENTED_EDGE ( 'NONE', *, *, #1774, .F. ) ;
#8978=ORIENTED_EDGE ( 'NONE', *, *, #363, .F. ) ;
#8993=ORIENTED_EDGE ( 'NONE', *, *, #9101, .F. ) ;
#9007=VECTOR ( 'NONE', #1221, 1000.000000000000000 ) ;
#9014=DIRECTION ( 'NONE',  ( 0.000000000000000000, -1.000000000000000000, 0.000000000000000000 ) ) ;
#9017=DIRECTION ( 'NONE',  ( -0.4712473909295827323, 0.000000000000000000, 0.8820010751365675583 ) ) ;
#9033=LINE ( 'NONE', #709, #6688 ) ;
#9043=ADVANCED_BREP_SHAPE_REPRESENTATION ( '', ( #1856, #2817 ), #6445 ) ;
#9049=DIRECTION ( 'NONE',  ( 0.000000000000000000, -1.000000000000000000, 0.000000000000000000 ) ) ;
#9052=DIRECTION ( 'NONE',  ( 0.000000000000000000, 1.000000000000000000, -0.000000000000000000 ) ) ;
#9066=DIRECTION ( 'NONE',  ( 0.000000000000000000, -1.000000000000000000, 0.000000000000000000 ) ) ;
#9067=VERTEX_POINT ( 'NONE', #486 ) ;
#9075=FACE_OUTER_BOUND ( 'NONE', #5323, .T. ) ;
#9081=LINE ( 'NONE', #3547, #6378 ) ;
#9083=EDGE_LOOP ( 'NONE', ( #4629, #4298, #2974, #2166 ) ) ;
#9088=CARTESIAN_POINT ( 'NONE',  ( -101.0297452788102817, -7.500000000000000000, -342.4231267849074811 ) ) ;
#9096=CARTESIAN_POINT ( 'NONE',  ( -46.74071243416547361, -7.500000000000000000, -414.3237589990478114 ) ) ;
#9101=EDGE_CURVE ( 'NONE', #3094, #4107, #592, .T. ) ;
#9120=CYLINDRICAL_SURFACE ( 'NONE', #1804, 5.000000000000008882 ) ;
#9124=CARTESIAN_POINT ( 'NONE',  ( -49.82771619714345235, -7.500000000000000000, -415.9731248673013511 ) ) ;
#9125=DIRECTION ( 'NONE',  ( -0.8820010751365676693, 0.000000000000000000, -0.4712473909295822883 ) ) ;
#9143=LINE ( 'NONE', #7478, #77 ) ;
#9153=UNCERTAINTY_MEASURE_WITH_UNIT (LENGTH_MEASURE( 1.000000000000000082E-05 ), #465, 'distance_accuracy_value', 'NONE');
#9180=DIRECTION ( 'NONE',  ( 0.000000000000000000, -1.000000000000000000, 0.000000000000000000 ) ) ;
#9182=AXIS2_PLACEMENT_3D ( 'NONE', #6385, #8052, #7359 ) ;
#9183=AXIS2_PLACEMENT_3D ( 'NONE', #10612, #4063, #2505 ) ;
#9213=CARTESIAN_POINT ( 'NONE',  ( -82.96626782902075092, -2.500000000000000000, -348.6449257547347997 ) ) ;
#9231=CARTESIAN_POINT ( 'NONE',  ( -81.08127826530241578, -2.500000000000000000, -352.1729300552810855 ) ) ;
#9234=DIRECTION ( 'NONE',  ( -0.8820010751365675583, 0.000000000000000000, -0.4712473909295827323 ) ) ;
#9252=ADVANCED_FACE ( 'NONE', ( #9666 ), #4082, .T. ) ;
#9257=DIRECTION ( 'NONE',  ( 0.8820010751365664481, 0.000000000000000000, 0.4712473909295847307 ) ) ;
#9270=PLANE ( 'NONE',  #4709 ) ;
#9275=AXIS2_PLACEMENT_3D ( 'NONE', #5543, #9049, #8884 ) ;
#9281=ORIENTED_EDGE ( 'NONE', *, *, #2353, .F. ) ;
#9294=DIRECTION ( 'NONE',  ( 0.8820010751365675583, 0.000000000000000000, 0.4712473909295827323 ) ) ;
#9316=VECTOR ( 'NONE', #1480, 1000.000000000000000 ) ;
#9321=CARTESIAN_POINT ( 'NONE',  ( -87.43676691142619006, -2.500000000000000000, -348.7659131681800773 ) ) ;
#9322=LINE ( 'NONE', #393, #5345 ) ;
#9335=FACE_OUTER_BOUND ( 'NONE', #9751, .T. ) ;
#9350=ORIENTED_EDGE ( 'NONE', *, *, #5835, .T. ) ;
#9352=AXIS2_PLACEMENT_3D ( 'NONE', #8333, #4204, #7579 ) ;
#9414=EDGE_CURVE ( 'NONE', #10567, #9606, #5227, .T. ) ;
#9422=CARTESIAN_POINT ( 'NONE',  ( -77.77979771402830522, -7.500000000000000000, -385.9384419754180158 ) ) ;
#9453=CARTESIAN_POINT ( 'NONE',  ( -86.86306229143158930, -2.500000000000000000, -370.6132103076870976 ) ) ;
#9456=DIRECTION ( 'NONE',  ( 0.8820010751365653379, 0.000000000000000000, 0.4712473909295871732 ) ) ;
#9463=DIRECTION ( 'NONE',  ( 0.000000000000000000, -1.000000000000000000, 0.000000000000000000 ) ) ;
#9501=VECTOR ( 'NONE', #9234, 1000.000000000000000 ) ;
#9502=ADVANCED_FACE ( 'NONE', ( #6647 ), #9120, .F. ) ;
#9509=CARTESIAN_POINT ( 'NONE',  ( -81.20226567874760804, -7.500000000000000000, -347.7024309728756748 ) ) ;
#9517=AXIS2_PLACEMENT_3D ( 'NONE', #5925, #132, #9052 ) ;
#9519=LINE ( 'NONE', #2209, #1593 ) ;
#9526=ORIENTED_EDGE ( 'NONE', *, *, #3251, .T. ) ;
#9538=DIRECTION ( 'NONE',  ( -0.8820010751365675583, 0.000000000000000000, -0.4712473909295827323 ) ) ;
#9552=EDGE_CURVE ( 'NONE', #3871, #7563, #4975, .T. ) ;
#9555=LINE ( 'NONE', #7732, #8531 ) ;
#9567=AXIS2_PLACEMENT_3D ( 'NONE', #324, #3648, #2089 ) ;
#9583=DIRECTION ( 'NONE',  ( 0.8820010751365675583, 0.000000000000000000, 0.4712473909295827323 ) ) ;
#9587=EDGE_LOOP ( 'NONE', ( #7918, #8646, #803, #8975 ) ) ;
#9592=LINE ( 'NONE', #3953, #7617 ) ;
#9593=( NAMED_UNIT ( * ) PLANE_ANGLE_UNIT ( ) SI_UNIT ( $, .RADIAN. ) );
#9600=VERTEX_POINT ( 'NONE', #5024 ) ;
#9606=VERTEX_POINT ( 'NONE', #1702 ) ;
#9616=EDGE_CURVE ( 'NONE', #1218, #8561, #8304, .T. ) ;
#9623=LINE ( 'NONE', #1514, #8055 ) ;
#9632=AXIS2_PLACEMENT_3D ( 'NONE', #6245, #3889, #5383 ) ;
#9666=FACE_OUTER_BOUND ( 'NONE', #9083, .T. ) ;
#9669=VECTOR ( 'NONE', #9538, 1000.000000000000000 ) ;
#9672=ORIENTED_EDGE ( 'NONE', *, *, #5752, .T. ) ;
#9696=ORIENTED_EDGE ( 'NONE', *, *, #8175, .F. ) ;
#9703=EDGE_CURVE ( 'NONE', #6862, #3094, #3731, .T. ) ;
#9710=VERTEX_POINT ( 'NONE', #2826 ) ;
#9729=FACE_OUTER_BOUND ( 'NONE', #7063, .T. ) ;
#9730=FACE_BOUND ( 'NONE', #5826, .T. ) ;
#9737=CARTESIAN_POINT ( 'NONE',  ( -83.90876261087991850, -2.500000000000000000, -346.8809236044617137 ) ) ;
#9741=CARTESIAN_POINT ( 'NONE',  ( -98.44423576012317767, -2.500000000000000000, -338.7741350709160315 ) ) ;
#9751=EDGE_LOOP ( 'NONE', ( #6982, #2689, #751, #3674 ) ) ;
#9762=ORIENTED_EDGE ( 'NONE', *, *, #10296, .T. ) ;
#9781=CIRCLE ( 'NONE', #1361, 4.000000000000009770 ) ;
#9782=VECTOR ( 'NONE', #8933, 1000.000000000000000 ) ;
#9808=ORIENTED_EDGE ( 'NONE', *, *, #7155, .T. ) ;
#9810=CARTESIAN_POINT ( 'NONE',  ( -87.43749534091338660, -2.500000000000000000, -367.8627987905216514 ) ) ;
#9817=ORIENTED_EDGE ( 'NONE', *, *, #1995, .F. ) ;
#9826=EDGE_CURVE ( 'NONE', #9710, #4191, #10371, .T. ) ;
#9856=CARTESIAN_POINT ( 'NONE',  ( -81.08127826530241578, -7.500000000000000000, -352.1729300552810855 ) ) ;
#9883=CARTESIAN_POINT ( 'NONE',  ( -86.86306229143158930, -7.500000000000000000, -370.6132103076870976 ) ) ;
#9892=ADVANCED_FACE ( 'NONE', ( #2657 ), #21, .T. ) ;
#9898=DIRECTION ( 'NONE',  ( 0.000000000000000000, 1.000000000000000000, -0.000000000000000000 ) ) ;
#9923=DIRECTION ( 'NONE',  ( 0.8820010751365664481, 0.000000000000000000, 0.4712473909295847307 ) ) ;
#9926=VECTOR ( 'NONE', #3588, 1000.000000000000000 ) ;
#9934=DIRECTION ( 'NONE',  ( -0.4712473909295827323, 0.000000000000000000, 0.8820010751365675583 ) ) ;
#9957=EDGE_CURVE ( 'NONE', #1052, #1738, #10277, .T. ) ;
#9962=ORIENTED_EDGE ( 'NONE', *, *, #4566, .T. ) ;
#9966=ORIENTED_EDGE ( 'NONE', *, *, #10481, .T. ) ;
#9969=ADVANCED_FACE ( 'NONE', ( #5320 ), #2914, .F. ) ;
#9977=ORIENTED_EDGE ( 'NONE', *, *, #6640, .F. ) ;
#9981=CARTESIAN_POINT ( 'NONE',  ( -77.67426137820133647, -2.500000000000000000, -345.8174414091573681 ) ) ;
#10004=DIRECTION ( 'NONE',  ( 0.4712473909295827323, 0.000000000000000000, -0.8820010751365675583 ) ) ;
#10029=EDGE_CURVE ( 'NONE', #5188, #8834, #7827, .T. ) ;
#10031=ORIENTED_EDGE ( 'NONE', *, *, #3927, .T. ) ;
#10041=DIRECTION ( 'NONE',  ( -0.8820010751365675583, 0.000000000000000000, -0.4712473909295827323 ) ) ;
#10060=LINE ( 'NONE', #1380, #5472 ) ;
#10070=ORIENTED_EDGE ( 'NONE', *, *, #8880, .F. ) ;
#10074=EDGE_CURVE ( 'NONE', #8561, #5927, #4072, .T. ) ;
#10091=CARTESIAN_POINT ( 'NONE',  ( -78.09771732525952359, -7.656480000000000175, -330.1706946207383453 ) ) ;
#10112=AXIS2_PLACEMENT_3D ( 'NONE', #7667, #1919, #2932 ) ;
#10118=ORIENTED_EDGE ( 'NONE', *, *, #7206, .T. ) ;
#10134=LINE ( 'NONE', #5445, #9669 ) ;
#10139=CARTESIAN_POINT ( 'NONE',  ( -85.25464975288055314, -2.500000000000000000, -378.3143625557585779 ) ) ;
#10148=VECTOR ( 'NONE', #916, 1000.000000000000000 ) ;
#10150=EDGE_CURVE ( 'NONE', #5927, #1373, #2460, .T. ) ;
#10151=DIRECTION ( 'NONE',  ( 0.9968876850330226080, 0.000000000000000000, -0.07883491250392217486 ) ) ;
#10169=FACE_OUTER_BOUND ( 'NONE', #5387, .T. ) ;
#10171=VERTEX_POINT ( 'NONE', #4338 ) ;
#10175=VECTOR ( 'NONE', #902, 1000.000000000000000 ) ;
#10190=CIRCLE ( 'NONE', #3845, 14.00000000000000888 ) ;
#10191=CARTESIAN_POINT ( 'NONE',  ( -79.04021210711869116, -7.500000000000000000, -328.4066924704651456 ) ) ;
#10192=EDGE_CURVE ( 'NONE', #4191, #8445, #7452, .T. ) ;
#10203=EDGE_LOOP ( 'NONE', ( #2561, #7080, #3734, #8028 ) ) ;
#10207=EDGE_CURVE ( 'NONE', #1519, #10171, #5135, .T. ) ;
#10208=DIRECTION ( 'NONE',  ( 0.000000000000000000, -1.000000000000000000, 0.000000000000000000 ) ) ;
#10212=AXIS2_PLACEMENT_3D ( 'NONE', #1701, #4974, #7448 ) ;
#10231=DIRECTION ( 'NONE',  ( 0.000000000000000000, 1.000000000000000000, -0.000000000000000000 ) ) ;
#10238=ORIENTED_EDGE ( 'NONE', *, *, #8908, .T. ) ;
#10244=DIRECTION ( 'NONE',  ( 0.000000000000000000, -1.000000000000000000, 0.000000000000000000 ) ) ;
#10246=ORIENTED_EDGE ( 'NONE', *, *, #7837, .F. ) ;
#10255=EDGE_LOOP ( 'NONE', ( #8513, #2340, #2084, #946 ) ) ;
#10277=LINE ( 'NONE', #6846, #1630 ) ;
#10290=CARTESIAN_POINT ( 'NONE',  ( -78.61675616006050404, -7.500000000000000000, -344.0534392588842252 ) ) ;
#10296=EDGE_CURVE ( 'NONE', #8202, #1052, #10134, .T. ) ;
#10298=VECTOR ( 'NONE', #4504, 1000.000000000000000 ) ;
#10304=ORIENTED_EDGE ( 'NONE', *, *, #5553, .T. ) ;
#10336=ORIENTED_EDGE ( 'NONE', *, *, #9703, .F. ) ;
#10341=LINE ( 'NONE', #1364, #9316 ) ;
#10342=ORIENTED_EDGE ( 'NONE', *, *, #4909, .F. ) ;
#10349=SURFACE_STYLE_USAGE ( .BOTH. , #4764 ) ;
#10359=FACE_BOUND ( 'NONE', #8189, .T. ) ;
#10371=CIRCLE ( 'NONE', #5917, 13.99999999999999645 ) ;
#10373=PLANE ( 'NONE',  #5794 ) ;
#10387=MECHANICAL_DESIGN_GEOMETRIC_PRESENTATION_REPRESENTATION('',(#4555),#8844);
#10396=( LENGTH_UNIT ( ) NAMED_UNIT ( * ) SI_UNIT ( .MILLI., .METRE. ) );
#10397=EDGE_CURVE ( 'NONE', #7778, #306, #1093, .T. ) ;
#10417=CARTESIAN_POINT ( 'NONE',  ( -78.09771732525952359, -2.500000000000000000, -330.1706946207383453 ) ) ;
#10419=PRODUCT_DEFINITION_SHAPE ( 'NONE', 'NONE',  #3305 ) ;
#10425=CARTESIAN_POINT ( 'NONE',  ( -102.0103468492230547, -2.500000000000000000, -289.6591388711787545 ) ) ;
#10460=VECTOR ( 'NONE', #7356, 1000.000000000000000 ) ;
#10481=EDGE_CURVE ( 'NONE', #7778, #6664, #7666, .T. ) ;
#10495=ORIENTED_EDGE ( 'NONE', *, *, #1671, .T. ) ;
#10501=CARTESIAN_POINT ( 'NONE',  ( -72.90663470096859555, -7.500000000000000000, -371.7168990827444190 ) ) ;
#10514=DIRECTION ( 'NONE',  ( -0.8820010751365653379, 0.000000000000000000, -0.4712473909295871732 ) ) ;
#10517=FACE_OUTER_BOUND ( 'NONE', #5299, .T. ) ;
#10545=AXIS2_PLACEMENT_3D ( 'NONE', #1128, #4506, #6936 ) ;
#10558=DIRECTION ( 'NONE',  ( -0.8820010751365675583, 0.000000000000000000, -0.4712473909295827323 ) ) ;
#10559=ORIENTED_EDGE ( 'NONE', *, *, #493, .T. ) ;
#10563=CARTESIAN_POINT ( 'NONE',  ( -72.90663470096859555, -7.500000000000000000, -371.7168990827444190 ) ) ;
#10567=VERTEX_POINT ( 'NONE', #7039 ) ;
#10593=CARTESIAN_POINT ( 'NONE',  ( -49.82771619714345235, -7.500000000000000000, -415.9731248673013511 ) ) ;
#10605=ORIENTED_EDGE ( 'NONE', *, *, #10029, .F. ) ;
#10610=DIRECTION ( 'NONE',  ( 0.000000000000000000, 1.000000000000000000, -0.000000000000000000 ) ) ;
#10611=ADVANCED_FACE ( 'NONE', ( #640, #10359, #8798, #1384 ), #2946, .T. ) ;
#10612=CARTESIAN_POINT ( 'NONE',  ( -82.14476046060677561, -2.366295999999999733, -345.9384288226025888 ) ) ;
#10616=EDGE_LOOP ( 'NONE', ( #778, #416, #9962, #10238 ) ) ;
#10617=DIRECTION ( 'NONE',  ( 0.000000000000000000, 1.000000000000000000, -0.000000000000000000 ) ) ;
ENDSEC;
END-ISO-10303-21;
